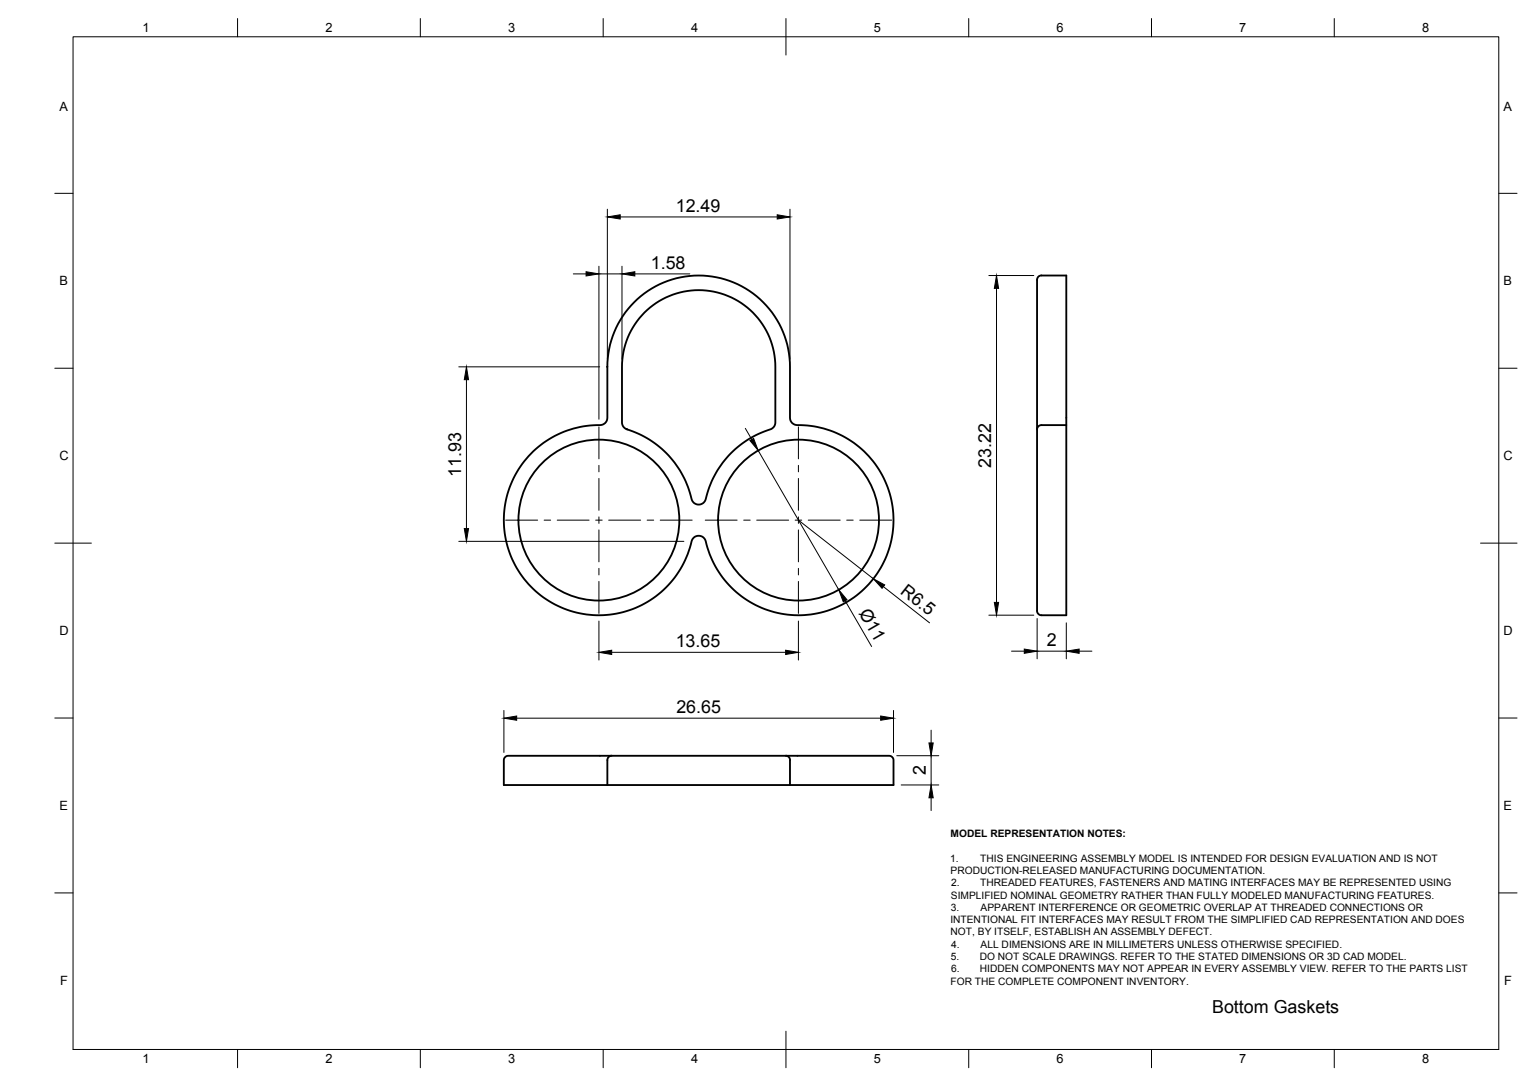
ISO-10303-21;
HEADER;
/* Generated by software containing ST-Developer
 * from STEP Tools, Inc. (www.steptools.com) 
 */

FILE_DESCRIPTION(
/* description */ ('STEP AP214'),
/* implementation_level */ '2;1');

FILE_NAME(
/* name */ 'Bottom Gaskets.step',
/* time_stamp */ '2026-10-06T00:19:40-07:00',
/* author */ (''),
/* organization */ (''),
/* preprocessor_version */ 'ST-DEVELOPER v20.2',
/* originating_system */ 'Autodesk Translation Framework v15.15.0.0',
/* authorisation */ '');

FILE_SCHEMA (('AUTOMOTIVE_DESIGN { 1 0 10303 214 3 1 1 }'));
ENDSEC;

DATA;
#10=MECHANICAL_DESIGN_GEOMETRIC_PRESENTATION_REPRESENTATION('',(#2066),#98302);
#118=TOROIDAL_SURFACE('',#34927,5.8,0.3);
#119=TOROIDAL_SURFACE('',#34931,5.8,0.3);
#569=ELLIPSE('',#34935,0.298848919318477,0.296905424707719);
#570=ELLIPSE('',#34936,0.298848892580485,0.296905360939291);
#571=ELLIPSE('',#34940,0.298848920090728,0.296905426638253);
#572=ELLIPSE('',#34941,0.29884889341624,0.296905361759044);
#573=ELLIPSE('',#34943,0.298848922260772,0.296905431625149);
#574=ELLIPSE('',#34945,0.298848920759339,0.296905428089205);
#575=ELLIPSE('',#34946,0.29884891933117,0.296905424743563);
#576=ELLIPSE('',#34947,0.298848915871755,0.296905416638318);
#577=ELLIPSE('',#34948,0.298848919843559,0.296905425953451);
#578=ELLIPSE('',#34949,0.298848891288725,0.296905359078035);
#579=ELLIPSE('',#34950,0.298848918410882,0.296905426718576);
#580=ELLIPSE('',#34951,0.298848922900226,0.296905433124464);
#581=ELLIPSE('',#34952,0.298848913927389,0.296905412076352);
#582=ELLIPSE('',#34953,0.298848922234263,0.296905431565699);
#583=ELLIPSE('',#34954,0.298848922236084,0.296905431557407);
#584=ELLIPSE('',#34956,0.298848891608559,0.296905359578392);
#585=ELLIPSE('',#34958,0.298848942238611,0.296905478386828);
#586=ELLIPSE('',#34959,0.298848922236084,0.296905431557407);
#1076=B_SPLINE_SURFACE_WITH_KNOTS('',5,5,((#72928,#72929,#72930,#72931,
#72932,#72933),(#72934,#72935,#72936,#72937,#72938,#72939),(#72940,#72941,
#72942,#72943,#72944,#72945),(#72946,#72947,#72948,#72949,#72950,#72951),
(#72952,#72953,#72954,#72955,#72956,#72957),(#72958,#72959,#72960,#72961,
#72962,#72963),(#72964,#72965,#72966,#72967,#72968,#72969),(#72970,#72971,
#72972,#72973,#72974,#72975),(#72976,#72977,#72978,#72979,#72980,#72981)),
 .UNSPECIFIED.,.F.,.F.,.F.,(6,3,6),(6,6),(0.546404786097,1.22269549144,
1.74380556781),(0.,0.3),.UNSPECIFIED.);
#1077=B_SPLINE_SURFACE_WITH_KNOTS('',5,1,((#72992,#72993),(#72994,#72995),
(#72996,#72997),(#72998,#72999),(#73000,#73001),(#73002,#73003)),
 .UNSPECIFIED.,.F.,.F.,.F.,(6,6),(2,2),(0.454732309483,1.10434989446),(0.,
0.204),.UNSPECIFIED.);
#1078=B_SPLINE_SURFACE_WITH_KNOTS('',5,5,((#73012,#73013,#73014,#73015,
#73016,#73017),(#73018,#73019,#73020,#73021,#73022,#73023),(#73024,#73025,
#73026,#73027,#73028,#73029),(#73030,#73031,#73032,#73033,#73034,#73035),
(#73036,#73037,#73038,#73039,#73040,#73041),(#73042,#73043,#73044,#73045,
#73046,#73047),(#73048,#73049,#73050,#73051,#73052,#73053),(#73054,#73055,
#73056,#73057,#73058,#73059),(#73060,#73061,#73062,#73063,#73064,#73065)),
 .UNSPECIFIED.,.F.,.F.,.F.,(6,3,6),(6,6),(6.80309055586,12.796423133,18.7900427979),
(0.,0.3),.UNSPECIFIED.);
#1079=B_SPLINE_SURFACE_WITH_KNOTS('',5,1,((#73074,#73075),(#73076,#73077),
(#73078,#73079),(#73080,#73081),(#73082,#73083),(#73084,#73085)),
 .UNSPECIFIED.,.F.,.F.,.F.,(6,6),(2,2),(5.9795921157,14.5218665667),(0.,
0.203999999999999),.UNSPECIFIED.);
#1080=B_SPLINE_SURFACE_WITH_KNOTS('',5,5,((#73087,#73088,#73089,#73090,
#73091,#73092),(#73093,#73094,#73095,#73096,#73097,#73098),(#73099,#73100,
#73101,#73102,#73103,#73104),(#73105,#73106,#73107,#73108,#73109,#73110),
(#73111,#73112,#73113,#73114,#73115,#73116),(#73117,#73118,#73119,#73120,
#73121,#73122),(#73123,#73124,#73125,#73126,#73127,#73128),(#73129,#73130,
#73131,#73132,#73133,#73134),(#73135,#73136,#73137,#73138,#73139,#73140)),
 .UNSPECIFIED.,.F.,.F.,.F.,(6,3,6),(6,6),(6.80400424079,13.5782854139,18.7904488943),
(0.,0.3),.UNSPECIFIED.);
#1081=B_SPLINE_SURFACE_WITH_KNOTS('',5,1,((#73201,#73202),(#73203,#73204),
(#73205,#73206),(#73207,#73208),(#73209,#73210),(#73211,#73212)),
 .UNSPECIFIED.,.F.,.F.,.F.,(6,6),(2,2),(5.9795921157,14.5218665667),(0.,
0.204),.UNSPECIFIED.);
#1082=B_SPLINE_SURFACE_WITH_KNOTS('',5,5,((#73220,#73221,#73222,#73223,
#73224,#73225),(#73226,#73227,#73228,#73229,#73230,#73231),(#73232,#73233,
#73234,#73235,#73236,#73237),(#73238,#73239,#73240,#73241,#73242,#73243),
(#73244,#73245,#73246,#73247,#73248,#73249),(#73250,#73251,#73252,#73253,
#73254,#73255),(#73256,#73257,#73258,#73259,#73260,#73261),(#73262,#73263,
#73264,#73265,#73266,#73267),(#73268,#73269,#73270,#73271,#73272,#73273)),
 .UNSPECIFIED.,.F.,.F.,.F.,(6,3,6),(6,6),(0.54640511867,1.22269582402,1.74380590038),
(0.,0.3),.UNSPECIFIED.);
#1083=B_SPLINE_SURFACE_WITH_KNOTS('',5,1,((#73282,#73283),(#73284,#73285),
(#73286,#73287),(#73288,#73289),(#73290,#73291),(#73292,#73293)),
 .UNSPECIFIED.,.F.,.F.,.F.,(6,6),(2,2),(0.454732309483,1.10434989446),(0.,
0.203999999999999),.UNSPECIFIED.);
#1084=B_SPLINE_SURFACE_WITH_KNOTS('',5,5,((#73295,#73296,#73297,#73298,
#73299,#73300),(#73301,#73302,#73303,#73304,#73305,#73306),(#73307,#73308,
#73309,#73310,#73311,#73312),(#73313,#73314,#73315,#73316,#73317,#73318),
(#73319,#73320,#73321,#73322,#73323,#73324),(#73325,#73326,#73327,#73328,
#73329,#73330),(#73331,#73332,#73333,#73334,#73335,#73336),(#73337,#73338,
#73339,#73340,#73341,#73342),(#73343,#73344,#73345,#73346,#73347,#73348)),
 .UNSPECIFIED.,.F.,.F.,.F.,(6,3,6),(6,6),(5.54615686267,10.8163068596,14.9229845471),
(0.,0.3),.UNSPECIFIED.);
#1085=B_SPLINE_SURFACE_WITH_KNOTS('',5,1,((#73357,#73358),(#73359,#73360),
(#73361,#73362),(#73363,#73364),(#73365,#73366),(#73367,#73368)),
 .UNSPECIFIED.,.F.,.F.,.F.,(6,6),(2,2),(4.82544286935,11.7189326827),(0.,
0.203999999999999),.UNSPECIFIED.);
#1086=B_SPLINE_SURFACE_WITH_KNOTS('',5,5,((#73370,#73371,#73372,#73373,
#73374,#73375),(#73376,#73377,#73378,#73379,#73380,#73381),(#73382,#73383,
#73384,#73385,#73386,#73387),(#73388,#73389,#73390,#73391,#73392,#73393),
(#73394,#73395,#73396,#73397,#73398,#73399),(#73400,#73401,#73402,#73403,
#73404,#73405),(#73406,#73407,#73408,#73409,#73410,#73411),(#73412,#73413,
#73414,#73415,#73416,#73417),(#73418,#73419,#73420,#73421,#73422,#73423)),
 .UNSPECIFIED.,.F.,.F.,.F.,(6,3,6),(6,6),(1.16471317114,2.5069575699,3.70327394785),
(0.,0.3),.UNSPECIFIED.);
#1087=B_SPLINE_SURFACE_WITH_KNOTS('',5,1,((#73478,#73479),(#73480,#73481),
(#73482,#73483),(#73484,#73485),(#73486,#73487),(#73488,#73489)),
 .UNSPECIFIED.,.F.,.F.,.F.,(6,6),(2,2),(1.04539060089,2.53880574503),(0.,
0.204),.UNSPECIFIED.);
#1088=B_SPLINE_SURFACE_WITH_KNOTS('',5,5,((#73491,#73492,#73493,#73494,
#73495,#73496),(#73497,#73498,#73499,#73500,#73501,#73502),(#73503,#73504,
#73505,#73506,#73507,#73508),(#73509,#73510,#73511,#73512,#73513,#73514),
(#73515,#73516,#73517,#73518,#73519,#73520),(#73521,#73522,#73523,#73524,
#73525,#73526),(#73527,#73528,#73529,#73530,#73531,#73532),(#73533,#73534,
#73535,#73536,#73537,#73538),(#73539,#73540,#73541,#73542,#73543,#73544)),
 .UNSPECIFIED.,.F.,.F.,.F.,(6,3,6),(6,6),(5.54628902772,10.8164390246,14.9231167121),
(0.,0.3),.UNSPECIFIED.);
#1089=B_SPLINE_SURFACE_WITH_KNOTS('',5,1,((#73551,#73552),(#73553,#73554),
(#73555,#73556),(#73557,#73558),(#73559,#73560),(#73561,#73562)),
 .UNSPECIFIED.,.F.,.F.,.F.,(6,6),(2,2),(4.82544286935,11.7189326827),(0.,
0.204),.UNSPECIFIED.);
#1090=B_SPLINE_SURFACE_WITH_KNOTS('',5,5,((#73563,#73564,#73565,#73566,
#73567,#73568),(#73569,#73570,#73571,#73572,#73573,#73574),(#73575,#73576,
#73577,#73578,#73579,#73580),(#73581,#73582,#73583,#73584,#73585,#73586),
(#73587,#73588,#73589,#73590,#73591,#73592),(#73593,#73594,#73595,#73596,
#73597,#73598),(#73599,#73600,#73601,#73602,#73603,#73604),(#73605,#73606,
#73607,#73608,#73609,#73610),(#73611,#73612,#73613,#73614,#73615,#73616)),
 .UNSPECIFIED.,.F.,.F.,.F.,(6,3,6),(6,6),(0.68208121853,1.52935115459,2.17454139046),
(0.,0.3),.UNSPECIFIED.);
#1091=B_SPLINE_SURFACE_WITH_KNOTS('',5,1,((#73627,#73628),(#73629,#73630),
(#73631,#73632),(#73633,#73634),(#73635,#73636),(#73637,#73638)),
 .UNSPECIFIED.,.F.,.F.,.F.,(6,6),(2,2),(0.574089330078,1.39421694447),(0.,
0.203999999999999),.UNSPECIFIED.);
#1092=B_SPLINE_SURFACE_WITH_KNOTS('',5,5,((#73641,#73642,#73643,#73644,
#73645,#73646),(#73647,#73648,#73649,#73650,#73651,#73652),(#73653,#73654,
#73655,#73656,#73657,#73658),(#73659,#73660,#73661,#73662,#73663,#73664),
(#73665,#73666,#73667,#73668,#73669,#73670),(#73671,#73672,#73673,#73674,
#73675,#73676),(#73677,#73678,#73679,#73680,#73681,#73682),(#73683,#73684,
#73685,#73686,#73687,#73688),(#73689,#73690,#73691,#73692,#73693,#73694),
(#73695,#73696,#73697,#73698,#73699,#73700),(#73701,#73702,#73703,#73704,
#73705,#73706),(#73707,#73708,#73709,#73710,#73711,#73712),(#73713,#73714,
#73715,#73716,#73717,#73718),(#73719,#73720,#73721,#73722,#73723,#73724),
(#73725,#73726,#73727,#73728,#73729,#73730)),.UNSPECIFIED.,.F.,.F.,.F.,
(6,3,3,3,6),(6,6),(13.4402611449,23.5689081291,33.6443676545,43.7196576595,
53.84849829),(0.,0.3),.UNSPECIFIED.);
#1093=B_SPLINE_SURFACE_WITH_KNOTS('',5,1,((#73748,#73749),(#73750,#73751),
(#73752,#73753),(#73754,#73755),(#73756,#73757),(#73758,#73759),(#73760,
#73761),(#73762,#73763),(#73764,#73765),(#73766,#73767),(#73768,#73769),
(#73770,#73771),(#73772,#73773),(#73774,#73775),(#73776,#73777)),
 .UNSPECIFIED.,.F.,.F.,.F.,(6,3,3,3,6),(2,2),(9.75975111992,17.2672519814,
24.7747528429,32.2822537043,39.7897545658),(0.,0.203999999999999),
 .UNSPECIFIED.);
#1094=B_SPLINE_SURFACE_WITH_KNOTS('',5,5,((#73779,#73780,#73781,#73782,
#73783,#73784),(#73785,#73786,#73787,#73788,#73789,#73790),(#73791,#73792,
#73793,#73794,#73795,#73796),(#73797,#73798,#73799,#73800,#73801,#73802),
(#73803,#73804,#73805,#73806,#73807,#73808),(#73809,#73810,#73811,#73812,
#73813,#73814),(#73815,#73816,#73817,#73818,#73819,#73820),(#73821,#73822,
#73823,#73824,#73825,#73826),(#73827,#73828,#73829,#73830,#73831,#73832)),
 .UNSPECIFIED.,.F.,.F.,.F.,(6,3,6),(6,6),(0.578957415869,1.29652194364,
1.84813902128),(0.,0.3),.UNSPECIFIED.);
#1095=B_SPLINE_SURFACE_WITH_KNOTS('',5,1,((#73841,#73842),(#73843,#73844),
(#73845,#73846),(#73847,#73848),(#73849,#73850),(#73851,#73852)),
 .UNSPECIFIED.,.F.,.F.,.F.,(6,6),(2,2),(0.48312294093,1.17329857083),(0.,
0.203999999999999),.UNSPECIFIED.);
#1096=B_SPLINE_SURFACE_WITH_KNOTS('',5,5,((#73854,#73855,#73856,#73857,
#73858,#73859),(#73860,#73861,#73862,#73863,#73864,#73865),(#73866,#73867,
#73868,#73869,#73870,#73871),(#73872,#73873,#73874,#73875,#73876,#73877),
(#73878,#73879,#73880,#73881,#73882,#73883),(#73884,#73885,#73886,#73887,
#73888,#73889),(#73890,#73891,#73892,#73893,#73894,#73895),(#73896,#73897,
#73898,#73899,#73900,#73901),(#73902,#73903,#73904,#73905,#73906,#73907)),
 .UNSPECIFIED.,.F.,.F.,.F.,(6,3,6),(6,6),(0.579418789984,1.29713059772,
1.84860050261),(0.,0.3),.UNSPECIFIED.);
#1097=B_SPLINE_SURFACE_WITH_KNOTS('',5,1,((#73916,#73917),(#73918,#73919),
(#73920,#73921),(#73922,#73923),(#73924,#73925),(#73926,#73927)),
 .UNSPECIFIED.,.F.,.F.,.F.,(6,6),(2,2),(0.48312294093,1.17329857083),(0.,
0.204),.UNSPECIFIED.);
#1098=B_SPLINE_SURFACE_WITH_KNOTS('',5,5,((#73929,#73930,#73931,#73932,
#73933,#73934),(#73935,#73936,#73937,#73938,#73939,#73940),(#73941,#73942,
#73943,#73944,#73945,#73946),(#73947,#73948,#73949,#73950,#73951,#73952),
(#73953,#73954,#73955,#73956,#73957,#73958),(#73959,#73960,#73961,#73962,
#73963,#73964),(#73965,#73966,#73967,#73968,#73969,#73970),(#73971,#73972,
#73973,#73974,#73975,#73976),(#73977,#73978,#73979,#73980,#73981,#73982),
(#73983,#73984,#73985,#73986,#73987,#73988),(#73989,#73990,#73991,#73992,
#73993,#73994),(#73995,#73996,#73997,#73998,#73999,#74000),(#74001,#74002,
#74003,#74004,#74005,#74006),(#74007,#74008,#74009,#74010,#74011,#74012),
(#74013,#74014,#74015,#74016,#74017,#74018)),.UNSPECIFIED.,.F.,.F.,.F.,
(6,3,3,3,6),(6,6),(13.4404181035,23.5157081046,33.5961540362,43.6766373031,
53.8487877185),(0.,0.3),.UNSPECIFIED.);
#1099=B_SPLINE_SURFACE_WITH_KNOTS('',5,1,((#74036,#74037),(#74038,#74039),
(#74040,#74041),(#74042,#74043),(#74044,#74045),(#74046,#74047),(#74048,
#74049),(#74050,#74051),(#74052,#74053),(#74054,#74055),(#74056,#74057),
(#74058,#74059),(#74060,#74061),(#74062,#74063),(#74064,#74065)),
 .UNSPECIFIED.,.F.,.F.,.F.,(6,3,3,3,6),(2,2),(9.75975111992,17.2672519814,
24.7747528429,32.2822537043,39.7897545658),(0.,0.203999999999999),
 .UNSPECIFIED.);
#1100=B_SPLINE_SURFACE_WITH_KNOTS('',5,5,((#74067,#74068,#74069,#74070,
#74071,#74072),(#74073,#74074,#74075,#74076,#74077,#74078),(#74079,#74080,
#74081,#74082,#74083,#74084),(#74085,#74086,#74087,#74088,#74089,#74090),
(#74091,#74092,#74093,#74094,#74095,#74096),(#74097,#74098,#74099,#74100,
#74101,#74102),(#74103,#74104,#74105,#74106,#74107,#74108),(#74109,#74110,
#74111,#74112,#74113,#74114),(#74115,#74116,#74117,#74118,#74119,#74120)),
 .UNSPECIFIED.,.F.,.F.,.F.,(6,3,6),(6,6),(0.682080632107,1.52935056816,
2.17454080403),(0.,0.3),.UNSPECIFIED.);
#1101=B_SPLINE_SURFACE_WITH_KNOTS('',5,1,((#74129,#74130),(#74131,#74132),
(#74133,#74134),(#74135,#74136),(#74137,#74138),(#74139,#74140)),
 .UNSPECIFIED.,.F.,.F.,.F.,(6,6),(2,2),(0.574089330078,1.39421694447),(0.,
0.203999999999999),.UNSPECIFIED.);
#1102=B_SPLINE_SURFACE_WITH_KNOTS('',5,5,((#74148,#74149,#74150,#74151,
#74152,#74153),(#74154,#74155,#74156,#74157,#74158,#74159),(#74160,#74161,
#74162,#74163,#74164,#74165),(#74166,#74167,#74168,#74169,#74170,#74171),
(#74172,#74173,#74174,#74175,#74176,#74177),(#74178,#74179,#74180,#74181,
#74182,#74183),(#74184,#74185,#74186,#74187,#74188,#74189),(#74190,#74191,
#74192,#74193,#74194,#74195),(#74196,#74197,#74198,#74199,#74200,#74201)),
 .UNSPECIFIED.,.F.,.F.,.F.,(6,3,6),(6,6),(8.03777014773,13.7697600959,21.5792812917),
(0.,0.3),.UNSPECIFIED.);
#1103=B_SPLINE_SURFACE_WITH_KNOTS('',5,1,((#74210,#74211),(#74212,#74213),
(#74214,#74215),(#74216,#74217),(#74218,#74219),(#74220,#74221)),
 .UNSPECIFIED.,.F.,.F.,.F.,(6,6),(2,2),(7.11986732816,17.2911063684),(0.,
0.204),.UNSPECIFIED.);
#1104=B_SPLINE_SURFACE_WITH_KNOTS('',5,5,((#74223,#74224,#74225,#74226,
#74227,#74228),(#74229,#74230,#74231,#74232,#74233,#74234),(#74235,#74236,
#74237,#74238,#74239,#74240),(#74241,#74242,#74243,#74244,#74245,#74246),
(#74247,#74248,#74249,#74250,#74251,#74252),(#74253,#74254,#74255,#74256,
#74257,#74258),(#74259,#74260,#74261,#74262,#74263,#74264),(#74265,#74266,
#74267,#74268,#74269,#74270),(#74271,#74272,#74273,#74274,#74275,#74276)),
 .UNSPECIFIED.,.F.,.F.,.F.,(6,3,6),(6,6),(8.03689290773,13.768506892,21.5784150656),
(0.,0.3),.UNSPECIFIED.);
#1105=B_SPLINE_SURFACE_WITH_KNOTS('',5,1,((#74285,#74286),(#74287,#74288),
(#74289,#74290),(#74291,#74292),(#74293,#74294),(#74295,#74296)),
 .UNSPECIFIED.,.F.,.F.,.F.,(6,6),(2,2),(7.11986732816,17.2911063684),(0.,
0.204000000000001),.UNSPECIFIED.);
#1268=FACE_BOUND('',#5840,.T.);
#1269=FACE_BOUND('',#5841,.T.);
#1270=FACE_BOUND('',#5842,.T.);
#1271=FACE_BOUND('',#5844,.T.);
#1272=FACE_BOUND('',#5845,.T.);
#1273=FACE_BOUND('',#5846,.T.);
#1591=B_SPLINE_CURVE_WITH_KNOTS('',3,(#71744,#71745,#71746,#71747,#71748,
#71749,#71750,#71751,#71752,#71753,#71754,#71755,#71756,#71757,#71758,#71759,
#71760,#71761,#71762,#71763,#71764,#71765,#71766,#71767,#71768,#71769,#71770,
#71771,#71772,#71773,#71774,#71775,#71776,#71777,#71778,#71779,#71780,#71781,
#71782,#71783,#71784,#71785,#71786,#71787,#71788,#71789,#71790,#71791,#71792,
#71793,#71794,#71795,#71796,#71797,#71798,#71799,#71800,#71801,#71802,#71803,
#71804,#71805,#71806,#71807,#71808,#71809,#71810,#71811,#71812,#71813,#71814,
#71815,#71816,#71817,#71818,#71819,#71820,#71821,#71822,#71823,#71824,#71825,
#71826,#71827,#71828,#71829,#71830,#71831,#71832,#71833,#71834,#71835,#71836,
#71837,#71838,#71839,#71840,#71841,#71842,#71843,#71844,#71845,#71846,#71847,
#71848,#71849,#71850,#71851,#71852,#71853,#71854,#71855,#71856,#71857,#71858,
#71859,#71860,#71861,#71862,#71863,#71864,#71865,#71866,#71867,#71868,#71869,
#71870,#71871,#71872,#71873,#71874,#71875,#71876,#71877,#71878,#71879,#71880,
#71881,#71882,#71883,#71884,#71885,#71886,#71887,#71888,#71889,#71890,#71891,
#71892,#71893,#71894,#71895,#71896,#71897,#71898,#71899,#71900,#71901,#71902,
#71903,#71904,#71905,#71906,#71907,#71908,#71909,#71910,#71911,#71912,#71913,
#71914,#71915,#71916,#71917,#71918),.UNSPECIFIED.,.F.,.F.,(4,3,3,3,3,3,
3,3,3,3,3,3,3,3,3,3,3,3,3,3,3,3,3,3,3,3,3,3,3,3,3,3,3,3,3,3,3,3,3,3,3,3,
3,3,3,3,3,3,3,3,3,3,3,3,3,3,3,3,4),(13.4402611449,13.5070964098,14.2468335688477,
14.9953689393349,15.7485030377147,16.5054819020246,17.2654067660921,18.0278474779116,
18.7905126436479,19.5517539434494,20.2095273779,20.9687643902614,21.7217135386243,
22.4703077255754,23.2116440479358,23.5689081291,24.3109067601058,25.0584792099068,
25.8110233837674,26.567773191108,27.3278022892921,28.1173729599431,28.8763863467288,
29.6393660388709,30.4006119455066,31.159144897169,31.9121345408492,32.6611814951464,
33.4038368880882,33.6443676545,34.3873867942773,35.135806909375,35.888999131998,
36.6461739203357,37.4063879012094,38.1955466209957,38.955487589057,39.7175566740638,
40.477710487504,41.2350068233562,41.9866165086,42.7342388949353,43.4754422745138,
43.7196576595,44.4613265079885,45.2089180014669,45.9618189072157,46.719235518721,
47.4801950110937,48.2678785133445,49.0291748631258,49.7910234685431,50.5510731777613,
51.3083055012999,52.0598033404119,52.8072294015329,53.5481010611059,53.7816630291,
53.84849829),.UNSPECIFIED.);
#1592=B_SPLINE_CURVE_WITH_KNOTS('',3,(#71920,#71921,#71922,#71923,#71924,
#71925,#71926,#71927,#71928,#71929,#71930,#71931,#71932,#71933,#71934,#71935,
#71936,#71937,#71938,#71939,#71940,#71941,#71942,#71943,#71944,#71945,#71946,
#71947,#71948,#71949,#71950,#71951,#71952,#71953,#71954,#71955,#71956,#71957,
#71958,#71959,#71960,#71961,#71962,#71963,#71964,#71965),.UNSPECIFIED.,
 .F.,.F.,(4,3,3,3,3,3,3,3,3,3,3,3,3,3,3,4),(0.68208121853,0.833285110291927,
0.893438704333,1.03975468193142,1.10556304245,1.23772138518436,1.36639838409707,
1.49153340548065,1.52935115459,1.66108737747387,1.74128259681,1.88383305622587,
1.95314956045,2.12228973264587,2.16523839884,2.17454139046),
 .UNSPECIFIED.);
#1593=B_SPLINE_CURVE_WITH_KNOTS('',3,(#71969,#71970,#71971,#71972,#71973,
#71974,#71975,#71976,#71977,#71978,#71979,#71980,#71981,#71982,#71983,#71984,
#71985,#71986,#71987,#71988,#71989,#71990,#71991,#71992,#71993,#71994,#71995,
#71996,#71997,#71998,#71999,#72000,#72001,#72002,#72003,#72004,#72005,#72006,
#72007,#72008,#72009,#72010,#72011,#72012,#72013,#72014,#72015,#72016,#72017,
#72018,#72019,#72020,#72021,#72022,#72023,#72024,#72025,#72026,#72027,#72028,
#72029),.UNSPECIFIED.,.F.,.F.,(4,3,3,3,3,3,3,3,3,3,3,3,3,3,3,3,3,3,3,3,
4),(8.03689290773,8.75334465576375,9.46923125712186,10.1895756567313,10.9140328563649,
11.6440191235026,12.3764813091007,13.1119708062231,13.768506892,14.5052662832091,
15.243807631294,15.9828982697244,16.7204464834581,17.4556667504414,18.1876202191916,
18.9154953869,19.6359475654664,20.3517214078531,21.0597384561033,21.5454531764,
21.5784150656),.UNSPECIFIED.);
#1594=B_SPLINE_CURVE_WITH_KNOTS('',3,(#72031,#72032,#72033,#72034,#72035,
#72036,#72037,#72038,#72039,#72040,#72041,#72042,#72043,#72044,#72045,#72046,
#72047,#72048,#72049,#72050,#72051,#72052,#72053,#72054,#72055,#72056,#72057,
#72058,#72059,#72060,#72061,#72062,#72063,#72064,#72065,#72066,#72067,#72068,
#72069,#72070,#72071,#72072,#72073,#72074,#72075,#72076,#72077,#72078,#72079,
#72080,#72081,#72082,#72083,#72084,#72085,#72086,#72087,#72088,#72089,#72090,
#72091),.UNSPECIFIED.,.F.,.F.,(4,3,3,3,3,3,3,3,3,3,3,3,3,3,3,3,3,3,3,3,
4),(8.03777014773,8.75426889125125,9.47001359609466,10.1902177205057,10.9145366724205,
11.6443893801527,12.3767202822979,13.1120832966385,13.7697600959,14.5065337688577,
15.2451024323911,15.9842354518727,16.7218509387113,17.4571540774596,18.1892052935327,
18.9171918235122,19.6377739811748,20.3536859093427,21.0618537376259,21.5465332101,
21.5792812917),.UNSPECIFIED.);
#1595=B_SPLINE_CURVE_WITH_KNOTS('',3,(#72095,#72096,#72097,#72098,#72099,
#72100,#72101,#72102,#72103,#72104,#72105,#72106,#72107,#72108,#72109,#72110,
#72111,#72112,#72113,#72114,#72115,#72116,#72117,#72118,#72119,#72120,#72121,
#72122,#72123,#72124,#72125,#72126,#72127,#72128,#72129,#72130,#72131,#72132,
#72133,#72134,#72135,#72136,#72137,#72138,#72139,#72140),.UNSPECIFIED.,
 .F.,.F.,(4,3,3,3,3,3,3,3,3,3,3,3,3,3,3,4),(0.682080632107,0.833188271917978,
0.893438117902,1.03975409805662,1.10556245601,1.23772079875137,1.36639779750311,
1.49153281928841,1.52935056816,1.66108679248608,1.74128201038,1.88383247191979,
1.95314897402,2.12228914750544,2.16523781241,2.17454080403),
 .UNSPECIFIED.);
#1596=B_SPLINE_CURVE_WITH_KNOTS('',3,(#72142,#72143,#72144,#72145,#72146,
#72147,#72148,#72149,#72150,#72151,#72152,#72153,#72154,#72155,#72156,#72157,
#72158,#72159,#72160,#72161,#72162,#72163,#72164,#72165,#72166,#72167,#72168,
#72169,#72170,#72171,#72172,#72173,#72174,#72175,#72176,#72177,#72178,#72179,
#72180,#72181,#72182,#72183,#72184,#72185,#72186,#72187,#72188,#72189,#72190,
#72191,#72192,#72193,#72194,#72195,#72196,#72197,#72198,#72199,#72200,#72201,
#72202,#72203,#72204,#72205,#72206,#72207,#72208,#72209,#72210,#72211,#72212,
#72213,#72214,#72215,#72216,#72217,#72218,#72219,#72220,#72221,#72222,#72223,
#72224,#72225,#72226,#72227,#72228,#72229,#72230,#72231,#72232,#72233,#72234,
#72235,#72236,#72237,#72238,#72239,#72240,#72241,#72242,#72243,#72244,#72245,
#72246,#72247,#72248,#72249,#72250,#72251,#72252,#72253,#72254,#72255,#72256,
#72257,#72258,#72259,#72260,#72261,#72262,#72263,#72264,#72265,#72266,#72267,
#72268,#72269,#72270,#72271,#72272,#72273,#72274,#72275,#72276,#72277,#72278,
#72279,#72280,#72281,#72282,#72283,#72284,#72285,#72286,#72287,#72288,#72289,
#72290,#72291,#72292,#72293,#72294,#72295,#72296,#72297,#72298,#72299,#72300,
#72301,#72302,#72303,#72304,#72305,#72306,#72307,#72308,#72309,#72310,#72311,
#72312,#72313),.UNSPECIFIED.,.F.,.F.,(4,3,3,3,3,3,3,3,3,3,3,3,3,3,3,3,3,
3,3,3,3,3,3,3,3,3,3,3,3,3,3,3,3,3,3,3,3,3,3,3,3,3,3,3,3,3,3,3,3,3,3,3,3,
3,3,3,3,4),(13.4404181035,14.1832469713423,14.9311788451456,15.6836632577811,
16.4417307823792,17.202055740606,17.9644513437534,18.4746549323,19.2374710902407,
19.9985815368466,20.7569924140862,21.509630605407,22.2582851244697,22.9999062408337,
23.5157081046,24.2597621045338,25.0092545320489,25.7635337985687,26.521784600003,
27.2830357102544,28.0721755009976,28.8305221896519,29.5929229482329,30.3533096498532,
31.1107361457363,31.8623257075202,32.6098454986528,33.3508338437457,33.5961540362,
34.3408789768401,35.0909966454356,35.8458336275569,36.6045522537918,37.3661601097332,
38.154969758904,38.8368239887457,39.599089755228,40.3593159984205,41.116556848427,
41.8678616724636,42.6150717427155,43.3555578410029,43.6766373031,44.4154372840554,
45.1632743442511,45.9157419950385,46.6741354613049,47.0360646138,47.7955806316773,
48.5576994151819,49.3198406379445,50.0808007763051,50.839431318698,51.5923911750364,
52.3413609598882,53.0826832013661,53.8176639786,53.8487877185),
 .UNSPECIFIED.);
#1597=B_SPLINE_CURVE_WITH_KNOTS('',3,(#72315,#72316,#72317,#72318,#72319,
#72320,#72321,#72322,#72323,#72324,#72325,#72326,#72327,#72328,#72329,#72330,
#72331,#72332,#72333,#72334,#72335,#72336,#72337,#72338,#72339,#72340,#72341,
#72342,#72343,#72344,#72345,#72346,#72347,#72348,#72349,#72350,#72351,#72352,
#72353,#72354),.UNSPECIFIED.,.F.,.F.,(4,3,3,3,3,3,3,3,3,3,3,3,3,4),(0.579418789984,
0.725653581578792,0.867122312367032,0.938068556291,1.07176782281773,1.11759224819,
1.24463101759673,1.29713059772,1.42927287787526,1.47665930895,1.61898723804258,
1.77132177608973,1.83573111331,1.84860050261),.UNSPECIFIED.);
#1598=B_SPLINE_CURVE_WITH_KNOTS('',3,(#72355,#72356,#72357,#72358,#72359,
#72360,#72361,#72362,#72363,#72364,#72365,#72366,#72367,#72368,#72369,#72370,
#72371,#72372,#72373,#72374,#72375,#72376,#72377,#72378,#72379,#72380,#72381,
#72382,#72383,#72384,#72385,#72386,#72387,#72388,#72389,#72390,#72391,#72392,
#72393,#72394),.UNSPECIFIED.,.F.,.F.,(4,3,3,3,3,3,3,3,3,3,3,3,3,4),(0.578957415869,
0.726935642898053,0.869358464457875,0.937512229109,1.07080769681197,1.19853817927595,
1.29652194364,1.42846234265899,1.4760627343,1.61769834304174,1.76863899687797,
1.83522042146,1.84649047214,1.84813902128),.UNSPECIFIED.);
#1599=B_SPLINE_CURVE_WITH_KNOTS('',3,(#72399,#72400,#72401,#72402,#72403,
#72404,#72405,#72406,#72407,#72408,#72409,#72410,#72411,#72412,#72413,#72414,
#72415,#72416,#72417,#72418,#72419,#72420,#72421,#72422,#72423,#72424,#72425,
#72426,#72427,#72428,#72429,#72430,#72431,#72432,#72433,#72434,#72435,#72436,
#72437,#72438),.UNSPECIFIED.,.F.,.F.,(4,3,3,3,3,3,3,3,3,3,3,3,3,4),(0.546404786097,
0.691378490918164,0.831851442486203,0.884338413692,1.0179759898933,1.05350843186,
1.1812184524978,1.22269549144,1.35451436280229,1.49122152065914,1.56106898317,
1.71044921676803,1.74092276094,1.74380556781),.UNSPECIFIED.);
#1600=B_SPLINE_CURVE_WITH_KNOTS('',3,(#72440,#72441,#72442,#72443,#72444,
#72445,#72446,#72447,#72448,#72449,#72450,#72451,#72452,#72453,#72454,#72455,
#72456,#72457,#72458,#72459,#72460,#72461,#72462,#72463,#72464,#72465,#72466,
#72467,#72468,#72469,#72470,#72471,#72472,#72473,#72474,#72475,#72476,#72477,
#72478,#72479,#72480,#72481,#72482),.UNSPECIFIED.,.F.,.F.,(4,3,3,3,3,3,
3,3,3,3,3,3,3,3,4),(5.54628902772,6.33044435630308,7.10830578793151,7.87994882881436,
8.64217889818713,9.39932532520428,10.1484181785832,10.8164390246,11.563804771993,
12.3219342993112,13.0975455758633,13.8843705850609,14.6884227142447,14.8537077686,
14.9231167121),.UNSPECIFIED.);
#1601=B_SPLINE_CURVE_WITH_KNOTS('',3,(#72484,#72485,#72486,#72487,#72488,
#72489,#72490,#72491,#72492,#72493,#72494,#72495,#72496,#72497,#72498,#72499,
#72500,#72501,#72502,#72503,#72504,#72505,#72506,#72507,#72508,#72509,#72510,
#72511,#72512,#72513,#72514,#72515,#72516,#72517,#72518,#72519,#72520,#72521,
#72522,#72523,#72524,#72525,#72526,#72527,#72528,#72529,#72530,#72531,#72532,
#72533,#72534,#72535,#72536,#72537,#72538,#72539,#72540,#72541,#72542,#72543,
#72544,#72545,#72546,#72547,#72548,#72549,#72550,#72551,#72552,#72553,#72554,
#72555,#72556,#72557,#72558,#72559),.UNSPECIFIED.,.F.,.F.,(4,3,3,3,3,3,
3,3,3,3,3,3,3,3,3,3,3,3,3,3,3,3,3,3,3,4),(1.16471317114,1.28955678457906,
1.34495894511,1.4697639644744,1.52520817925,1.65292971547884,1.76872520496,
1.90134001405299,2.0346343138382,2.13573896786,2.26681625793335,2.39531374620892,
2.5069575699,2.6339538548235,2.76351336933892,2.87774629091,3.00835142684093,
3.12090556789,3.24957903139955,3.30443948601,3.43081011387895,3.48797183209,
3.613503668297,3.67393178216,3.69717524887,3.70327394785),.UNSPECIFIED.);
#1602=B_SPLINE_CURVE_WITH_KNOTS('',3,(#72561,#72562,#72563,#72564,#72565,
#72566,#72567,#72568,#72569,#72570,#72571,#72572,#72573,#72574,#72575,#72576,
#72577,#72578,#72579,#72580,#72581,#72582,#72583,#72584,#72585,#72586,#72587,
#72588,#72589,#72590,#72591,#72592,#72593,#72594,#72595,#72596,#72597,#72598,
#72599,#72600,#72601,#72602,#72603,#72604,#72605,#72606),.UNSPECIFIED.,
 .F.,.F.,(4,3,3,3,3,3,3,3,3,3,3,3,3,3,3,4),(5.54615686267,6.33030620256032,
7.10816058979279,7.87979597471841,8.64201814773229,9.39915688584315,10.1482427247414,
10.8163068596,11.5638110745412,12.3220901845671,13.098030834098,13.8852098339371,
14.4040971905186,14.6843128354211,14.8776367646747,14.9229845471),
 .UNSPECIFIED.);
#1603=B_SPLINE_CURVE_WITH_KNOTS('',3,(#72608,#72609,#72610,#72611,#72612,
#72613,#72614,#72615,#72616,#72617,#72618,#72619,#72620,#72621,#72622,#72623,
#72624,#72625,#72626,#72627,#72628,#72629,#72630,#72631,#72632,#72633,#72634,
#72635,#72636,#72637,#72638,#72639,#72640,#72641,#72642,#72643,#72644),
 .UNSPECIFIED.,.F.,.F.,(4,3,3,3,3,3,3,3,3,3,3,3,4),(0.54640511867,0.69038189628902,
0.831066058366692,0.965751341507189,1.05350876443,1.1812187883191,1.22269582402,
1.35451469641816,1.49122185483681,1.56106931574,1.71044954193083,1.74092309351,
1.74380590038),.UNSPECIFIED.);
#1604=B_SPLINE_CURVE_WITH_KNOTS('',3,(#72648,#72649,#72650,#72651,#72652,
#72653,#72654,#72655,#72656,#72657,#72658,#72659,#72660,#72661,#72662,#72663,
#72664,#72665,#72666,#72667,#72668,#72669,#72670,#72671,#72672,#72673,#72674,
#72675,#72676,#72677,#72678,#72679,#72680,#72681,#72682,#72683,#72684,#72685,
#72686,#72687,#72688,#72689,#72690,#72691,#72692,#72693,#72694,#72695,#72696,
#72697,#72698,#72699,#72700,#72701,#72702,#72703,#72704,#72705,#72706,#72707,
#72708),.UNSPECIFIED.,.F.,.F.,(4,3,3,3,3,3,3,3,3,3,3,3,3,3,3,3,3,3,3,3,
4),(6.80400424079,7.43551608490868,8.07296241255818,8.71878211416777,9.36915323230095,
10.0253311081077,10.185707897,10.847851527524,11.530459999118,12.1974538393883,
12.8878696266442,13.5782854139,14.2435799397826,14.905962344532,15.5649203367182,
16.2200258486319,16.8684640346437,17.5129910403709,18.1507928771493,18.7732643273,
18.7904488943),.UNSPECIFIED.);
#1605=B_SPLINE_CURVE_WITH_KNOTS('',3,(#72709,#72710,#72711,#72712,#72713,
#72714,#72715,#72716,#72717,#72718,#72719,#72720,#72721,#72722,#72723,#72724,
#72725,#72726,#72727,#72728,#72729,#72730,#72731,#72732,#72733,#72734,#72735,
#72736,#72737,#72738,#72739,#72740,#72741,#72742,#72743,#72744,#72745,#72746,
#72747,#72748,#72749,#72750,#72751,#72752,#72753,#72754,#72755,#72756,#72757,
#72758,#72759,#72760,#72761,#72762,#72763,#72764,#72765,#72766,#72767,#72768,
#72769,#72770,#72771,#72772,#72773,#72774,#72775),.UNSPECIFIED.,.F.,.F.,
(4,3,3,3,3,3,3,3,3,3,3,3,3,3,3,3,3,3,3,3,3,3,4),(6.80309055586,6.83920298432,
7.47379817923227,8.13912629845323,8.78763073366937,9.44086248718233,10.0984392541387,
10.7729352238541,11.4388498023207,12.1176364676603,12.796423133,13.4656868144225,
14.132263549812,14.7961195641698,15.4565492516297,16.112959614828,16.782230410596,
17.4269097691535,18.0671355216093,18.4285891597547,18.6334246721777,18.7701216625788,
18.7900427979),.UNSPECIFIED.);
#1606=B_SPLINE_CURVE_WITH_KNOTS('',5,(#72783,#72784,#72785,#72786,#72787,
#72788),.UNSPECIFIED.,.F.,.F.,(6,6),(-0.791045523784,0.),.UNSPECIFIED.);
#1607=B_SPLINE_CURVE_WITH_KNOTS('',5,(#72790,#72791,#72792,#72793,#72794,
#72795,#72796,#72797,#72798,#72799,#72800,#72801,#72802,#72803,#72804),
 .UNSPECIFIED.,.F.,.F.,(6,3,3,3,6),(-30.0305934991,-22.7207065053,-15.4108195114,
-8.10093251761,-0.791045523784),.UNSPECIFIED.);
#1608=B_SPLINE_CURVE_WITH_KNOTS('',5,(#72806,#72807,#72808,#72809,#72810,
#72811),.UNSPECIFIED.,.F.,.F.,(6,6),(-30.70334581,-30.0305934991),
 .UNSPECIFIED.);
#1609=B_SPLINE_CURVE_WITH_KNOTS('',5,(#72813,#72814,#72815,#72816,#72817,
#72818),.UNSPECIFIED.,.F.,.F.,(6,6),(-31.3760981209,-30.70334581),
 .UNSPECIFIED.);
#1610=B_SPLINE_CURVE_WITH_KNOTS('',5,(#72820,#72821,#72822,#72823,#72824,
#72825,#72826,#72827,#72828,#72829,#72830,#72831,#72832,#72833,#72834),
 .UNSPECIFIED.,.F.,.F.,(6,3,3,3,6),(-60.6156460962,-53.3057591024,-45.9958721086,
-38.6859851147,-31.3760981209),.UNSPECIFIED.);
#1611=B_SPLINE_CURVE_WITH_KNOTS('',5,(#72836,#72837,#72838,#72839,#72840,
#72841),.UNSPECIFIED.,.F.,.F.,(6,6),(-61.40669162,-60.6156460962),
 .UNSPECIFIED.);
#1612=B_SPLINE_CURVE_WITH_KNOTS('',5,(#72845,#72846,#72847,#72848,#72849,
#72850),.UNSPECIFIED.,.F.,.F.,(6,6),(-74.6958207115,-64.888669513),
 .UNSPECIFIED.);
#1613=B_SPLINE_CURVE_WITH_KNOTS('',5,(#72852,#72853,#72854,#72855,#72856,
#72857),.UNSPECIFIED.,.F.,.F.,(6,6),(-84.5029719101,-74.6958207115),
 .UNSPECIFIED.);
#1614=B_SPLINE_CURVE_WITH_KNOTS('',5,(#72865,#72866,#72867,#72868,#72869,
#72870),.UNSPECIFIED.,.F.,.F.,(6,6),(0.,0.634618899121),.UNSPECIFIED.);
#1615=B_SPLINE_CURVE_WITH_KNOTS('',5,(#72874,#72875,#72876,#72877,#72878,
#72879),.UNSPECIFIED.,.F.,.F.,(6,6),(4.43202703274,12.6683819045),
 .UNSPECIFIED.);
#1616=B_SPLINE_CURVE_WITH_KNOTS('',5,(#72881,#72882,#72883,#72884,#72885,
#72886),.UNSPECIFIED.,.F.,.F.,(6,6),(12.6683819045,20.9047367763),
 .UNSPECIFIED.);
#1617=B_SPLINE_CURVE_WITH_KNOTS('',5,(#72890,#72891,#72892,#72893,#72894,
#72895),.UNSPECIFIED.,.F.,.F.,(6,6),(24.7021449099,25.336763809),
 .UNSPECIFIED.);
#1618=B_SPLINE_CURVE_WITH_KNOTS('',5,(#72897,#72898,#72899,#72900,#72901,
#72902),.UNSPECIFIED.,.F.,.F.,(6,6),(25.336763809,32.1215862286),
 .UNSPECIFIED.);
#1619=B_SPLINE_CURVE_WITH_KNOTS('',5,(#72904,#72905,#72906,#72907,#72908,
#72909),.UNSPECIFIED.,.F.,.F.,(6,6),(32.1215862286,33.4669635909),
 .UNSPECIFIED.);
#1620=B_SPLINE_CURVE_WITH_KNOTS('',5,(#72910,#72911,#72912,#72913,#72914,
#72915),.UNSPECIFIED.,.F.,.F.,(6,6),(33.4669635909,40.2517860105),
 .UNSPECIFIED.);
#1621=B_SPLINE_CURVE_WITH_KNOTS('',5,(#72986,#72987,#72988,#72989,#72990,
#72991),.UNSPECIFIED.,.F.,.F.,(6,6),(0.,1.),.UNSPECIFIED.);
#1622=B_SPLINE_CURVE_WITH_KNOTS('',5,(#73068,#73069,#73070,#73071,#73072,
#73073),.UNSPECIFIED.,.F.,.F.,(6,6),(4.43202703274,12.6683819045),
 .UNSPECIFIED.);
#1623=B_SPLINE_CURVE_WITH_KNOTS('',3,(#73143,#73144,#73145,#73146,#73147,
#73148,#73149,#73150,#73151,#73152,#73153,#73154,#73155,#73156,#73157,#73158,
#73159,#73160,#73161,#73162,#73163,#73164,#73165,#73166,#73167,#73168,#73169,
#73170,#73171,#73172,#73173,#73174,#73175,#73176,#73177,#73178,#73179,#73180,
#73181,#73182,#73183,#73184,#73185,#73186,#73187,#73188,#73189,#73190,#73191,
#73192,#73193,#73194,#73195,#73196,#73197,#73198,#73199,#73200),
 .UNSPECIFIED.,.F.,.F.,(4,3,3,3,3,3,3,3,3,3,3,3,3,3,3,3,3,3,3,4),(12.6683819045,
13.1106199615824,13.5570304890591,14.0277809275642,14.4835378398279,14.9420145479918,
15.4026526010081,15.882747950031,16.3457775995096,16.8085437495859,17.2700435239617,
17.3230339970997,17.7823518959161,18.2417043637307,18.7003769570558,19.1576865479113,
19.6116903525143,20.0633375875012,20.5105511785383,20.9047367763),
 .UNSPECIFIED.);
#1624=B_SPLINE_CURVE_WITH_KNOTS('',5,(#73276,#73277,#73278,#73279,#73280,
#73281),.UNSPECIFIED.,.F.,.F.,(6,6),(0.,1.),.UNSPECIFIED.);
#1625=B_SPLINE_CURVE_WITH_KNOTS('',5,(#73351,#73352,#73353,#73354,#73355,
#73356),.UNSPECIFIED.,.F.,.F.,(6,6),(25.336763809,32.1215862286),
 .UNSPECIFIED.);
#1626=B_SPLINE_CURVE_WITH_KNOTS('',3,(#73426,#73427,#73428,#73429,#73430,
#73431,#73432,#73433,#73434,#73435,#73436,#73437,#73438,#73439,#73440,#73441,
#73442,#73443,#73444,#73445,#73446,#73447,#73448,#73449,#73450,#73451,#73452,
#73453,#73454,#73455,#73456,#73457,#73458,#73459,#73460,#73461,#73462,#73463,
#73464,#73465,#73466,#73467,#73468,#73469,#73470,#73471,#73472,#73473,#73474,
#73475,#73476,#73477),.UNSPECIFIED.,.F.,.F.,(4,3,3,3,3,3,3,3,3,3,3,3,3,
3,3,3,3,4),(0.,0.0568525693849193,0.115818688059534,0.173763369030792,0.232053865677185,
0.290632777510717,0.350119962828498,0.409067978904654,0.468824748843247,
0.528581518781839,0.587508828934109,0.646482285375474,0.705424215615768,
0.764242216553829,0.823181662415371,0.881380292059083,0.940690146029541,
1.),.UNSPECIFIED.);
#1627=B_SPLINE_CURVE_WITH_KNOTS('',5,(#73545,#73546,#73547,#73548,#73549,
#73550),.UNSPECIFIED.,.F.,.F.,(6,6),(33.4669635909,40.2517860105),
 .UNSPECIFIED.);
#1628=B_SPLINE_CURVE_WITH_KNOTS('',5,(#73620,#73621,#73622,#73623,#73624,
#73625),.UNSPECIFIED.,.F.,.F.,(6,6),(-1.39421694447,-0.574089330078),
 .UNSPECIFIED.);
#1629=B_SPLINE_CURVE_WITH_KNOTS('',5,(#73733,#73734,#73735,#73736,#73737,
#73738,#73739,#73740,#73741,#73742,#73743,#73744,#73745,#73746,#73747),
 .UNSPECIFIED.,.F.,.F.,(6,3,3,3,6),(-39.7897545658,-32.2822537043,-24.7747528429,
-17.2672519814,-9.75975111992),.UNSPECIFIED.);
#1630=B_SPLINE_CURVE_WITH_KNOTS('',5,(#73835,#73836,#73837,#73838,#73839,
#73840),.UNSPECIFIED.,.F.,.F.,(6,6),(-0.336376155459,0.336376155459),
 .UNSPECIFIED.);
#1631=B_SPLINE_CURVE_WITH_KNOTS('',5,(#73910,#73911,#73912,#73913,#73914,
#73915),.UNSPECIFIED.,.F.,.F.,(6,6),(-0.336376155459,0.336376155459),
 .UNSPECIFIED.);
#1632=B_SPLINE_CURVE_WITH_KNOTS('',5,(#74021,#74022,#74023,#74024,#74025,
#74026,#74027,#74028,#74029,#74030,#74031,#74032,#74033,#74034,#74035),
 .UNSPECIFIED.,.F.,.F.,(6,3,3,3,6),(-39.7897545658,-32.2822537043,-24.7747528429,
-17.2672519814,-9.75975111992),.UNSPECIFIED.);
#1633=B_SPLINE_CURVE_WITH_KNOTS('',5,(#74123,#74124,#74125,#74126,#74127,
#74128),.UNSPECIFIED.,.F.,.F.,(6,6),(-1.39421694447,-0.574089330078),
 .UNSPECIFIED.);
#1634=B_SPLINE_CURVE_WITH_KNOTS('',5,(#74204,#74205,#74206,#74207,#74208,
#74209),.UNSPECIFIED.,.F.,.F.,(6,6),(-4.90357559929,4.90357559929),
 .UNSPECIFIED.);
#1635=B_SPLINE_CURVE_WITH_KNOTS('',5,(#74279,#74280,#74281,#74282,#74283,
#74284),.UNSPECIFIED.,.F.,.F.,(6,6),(-4.90357559929,4.90357559929),
 .UNSPECIFIED.);
#2046=SHAPE_REPRESENTATION_RELATIONSHIP('SRR','None',#98343,#2056);
#2056=ADVANCED_BREP_SHAPE_REPRESENTATION('',(#2076),#98295);
#2066=STYLED_ITEM('',(#98399),#2076);
#2076=MANIFOLD_SOLID_BREP('Body1',#34170);
#2125=PLANE('',#34921);
#2126=PLANE('',#34924);
#2127=PLANE('',#34939);
#2128=PLANE('',#34944);
#2129=PLANE('',#34957);
#2130=PLANE('',#34961);
#2614=CYLINDRICAL_SURFACE('',#34930,5.5);
#2615=CYLINDRICAL_SURFACE('',#34934,5.5);
#2616=CYLINDRICAL_SURFACE('',#34937,0.3);
#2617=CYLINDRICAL_SURFACE('',#34942,0.3);
#2618=CYLINDRICAL_SURFACE('',#34955,0.3);
#2619=CYLINDRICAL_SURFACE('',#34960,0.3);
#3685=FACE_OUTER_BOUND('',#5839,.T.);
#3686=FACE_OUTER_BOUND('',#5843,.T.);
#3687=FACE_OUTER_BOUND('',#5847,.T.);
#3688=FACE_OUTER_BOUND('',#5848,.T.);
#3689=FACE_OUTER_BOUND('',#5849,.T.);
#3690=FACE_OUTER_BOUND('',#5850,.T.);
#3691=FACE_OUTER_BOUND('',#5851,.T.);
#3692=FACE_OUTER_BOUND('',#5852,.T.);
#3693=FACE_OUTER_BOUND('',#5853,.T.);
#3694=FACE_OUTER_BOUND('',#5854,.T.);
#3695=FACE_OUTER_BOUND('',#5855,.T.);
#3696=FACE_OUTER_BOUND('',#5856,.T.);
#3697=FACE_OUTER_BOUND('',#5857,.T.);
#3698=FACE_OUTER_BOUND('',#5858,.T.);
#3699=FACE_OUTER_BOUND('',#5859,.T.);
#3700=FACE_OUTER_BOUND('',#5860,.T.);
#3701=FACE_OUTER_BOUND('',#5861,.T.);
#3702=FACE_OUTER_BOUND('',#5862,.T.);
#3703=FACE_OUTER_BOUND('',#5863,.T.);
#3704=FACE_OUTER_BOUND('',#5864,.T.);
#3705=FACE_OUTER_BOUND('',#5865,.T.);
#3706=FACE_OUTER_BOUND('',#5866,.T.);
#3707=FACE_OUTER_BOUND('',#5867,.T.);
#3708=FACE_OUTER_BOUND('',#5868,.T.);
#3709=FACE_OUTER_BOUND('',#5869,.T.);
#3710=FACE_OUTER_BOUND('',#5870,.T.);
#3711=FACE_OUTER_BOUND('',#5871,.T.);
#3712=FACE_OUTER_BOUND('',#5872,.T.);
#3713=FACE_OUTER_BOUND('',#5873,.T.);
#3714=FACE_OUTER_BOUND('',#5874,.T.);
#3715=FACE_OUTER_BOUND('',#5875,.T.);
#3716=FACE_OUTER_BOUND('',#5876,.T.);
#3717=FACE_OUTER_BOUND('',#5877,.T.);
#3718=FACE_OUTER_BOUND('',#5878,.T.);
#3719=FACE_OUTER_BOUND('',#5879,.T.);
#3720=FACE_OUTER_BOUND('',#5880,.T.);
#3721=FACE_OUTER_BOUND('',#5881,.T.);
#3722=FACE_OUTER_BOUND('',#5882,.T.);
#3723=FACE_OUTER_BOUND('',#5883,.T.);
#3724=FACE_OUTER_BOUND('',#5884,.T.);
#3725=FACE_OUTER_BOUND('',#5885,.T.);
#3726=FACE_OUTER_BOUND('',#5886,.T.);
#3727=FACE_OUTER_BOUND('',#5887,.T.);
#3728=FACE_OUTER_BOUND('',#5888,.T.);
#5839=EDGE_LOOP('',(#23727,#23728,#23729,#23730,#23731,#23732,#23733,#23734,
#23735,#23736));
#5840=EDGE_LOOP('',(#23737,#23738,#23739,#23740,#23741,#23742,#23743,#23744,
#23745));
#5841=EDGE_LOOP('',(#23746));
#5842=EDGE_LOOP('',(#23747));
#5843=EDGE_LOOP('',(#23748,#23749,#23750,#23751,#23752,#23753,#23754,#23755,
#23756,#23757));
#5844=EDGE_LOOP('',(#23758));
#5845=EDGE_LOOP('',(#23759));
#5846=EDGE_LOOP('',(#23760,#23761,#23762,#23763,#23764,#23765,#23766,#23767,
#23768));
#5847=EDGE_LOOP('',(#23769,#23770,#23771,#23772));
#5848=EDGE_LOOP('',(#23773,#23774,#23775,#23776));
#5849=EDGE_LOOP('',(#23777,#23778,#23779,#23780));
#5850=EDGE_LOOP('',(#23781,#23782,#23783,#23784));
#5851=EDGE_LOOP('',(#23785,#23786,#23787,#23788));
#5852=EDGE_LOOP('',(#23789,#23790,#23791,#23792));
#5853=EDGE_LOOP('',(#23793,#23794,#23795,#23796));
#5854=EDGE_LOOP('',(#23797,#23798,#23799,#23800));
#5855=EDGE_LOOP('',(#23801,#23802,#23803,#23804));
#5856=EDGE_LOOP('',(#23805,#23806,#23807,#23808));
#5857=EDGE_LOOP('',(#23809,#23810,#23811,#23812));
#5858=EDGE_LOOP('',(#23813,#23814,#23815,#23816));
#5859=EDGE_LOOP('',(#23817,#23818,#23819,#23820));
#5860=EDGE_LOOP('',(#23821,#23822,#23823,#23824));
#5861=EDGE_LOOP('',(#23825,#23826,#23827,#23828));
#5862=EDGE_LOOP('',(#23829,#23830,#23831,#23832));
#5863=EDGE_LOOP('',(#23833,#23834,#23835,#23836));
#5864=EDGE_LOOP('',(#23837,#23838,#23839,#23840));
#5865=EDGE_LOOP('',(#23841,#23842,#23843,#23844));
#5866=EDGE_LOOP('',(#23845,#23846,#23847,#23848));
#5867=EDGE_LOOP('',(#23849,#23850,#23851,#23852));
#5868=EDGE_LOOP('',(#23853,#23854,#23855,#23856));
#5869=EDGE_LOOP('',(#23857,#23858,#23859,#23860));
#5870=EDGE_LOOP('',(#23861,#23862,#23863,#23864));
#5871=EDGE_LOOP('',(#23865,#23866,#23867,#23868));
#5872=EDGE_LOOP('',(#23869,#23870,#23871,#23872));
#5873=EDGE_LOOP('',(#23873,#23874,#23875,#23876));
#5874=EDGE_LOOP('',(#23877,#23878,#23879,#23880));
#5875=EDGE_LOOP('',(#23881,#23882,#23883,#23884));
#5876=EDGE_LOOP('',(#23885,#23886,#23887,#23888));
#5877=EDGE_LOOP('',(#23889,#23890,#23891,#23892));
#5878=EDGE_LOOP('',(#23893,#23894,#23895,#23896));
#5879=EDGE_LOOP('',(#23897,#23898,#23899,#23900));
#5880=EDGE_LOOP('',(#23901,#23902,#23903,#23904));
#5881=EDGE_LOOP('',(#23905,#23906,#23907,#23908));
#5882=EDGE_LOOP('',(#23909,#23910,#23911,#23912));
#5883=EDGE_LOOP('',(#23913,#23914,#23915,#23916));
#5884=EDGE_LOOP('',(#23917,#23918,#23919,#23920));
#5885=EDGE_LOOP('',(#23921,#23922,#23923,#23924));
#5886=EDGE_LOOP('',(#23925,#23926,#23927,#23928));
#5887=EDGE_LOOP('',(#23929,#23930,#23931,#23932));
#5888=EDGE_LOOP('',(#23933,#23934,#23935,#23936));
#7916=LINE('',#71967,#9756);
#7917=LINE('',#72093,#9757);
#7918=LINE('',#72397,#9758);
#7919=LINE('',#72646,#9759);
#7920=LINE('',#72843,#9760);
#7921=LINE('',#72858,#9761);
#7922=LINE('',#72872,#9762);
#7923=LINE('',#72888,#9763);
#7924=LINE('',#72921,#9764);
#7925=LINE('',#72927,#9765);
#7926=LINE('',#73004,#9766);
#7927=LINE('',#73005,#9767);
#7928=LINE('',#73009,#9768);
#7929=LINE('',#73011,#9769);
#7930=LINE('',#73086,#9770);
#7931=LINE('',#73213,#9771);
#7932=LINE('',#73217,#9772);
#7933=LINE('',#73219,#9773);
#7934=LINE('',#73294,#9774);
#7935=LINE('',#73369,#9775);
#7936=LINE('',#73490,#9776);
#7937=LINE('',#73639,#9777);
#7938=LINE('',#73640,#9778);
#7939=LINE('',#73778,#9779);
#7940=LINE('',#73853,#9780);
#7941=LINE('',#73928,#9781);
#7942=LINE('',#74066,#9782);
#7943=LINE('',#74141,#9783);
#7944=LINE('',#74145,#9784);
#7945=LINE('',#74147,#9785);
#7946=LINE('',#74222,#9786);
#7947=LINE('',#74297,#9787);
#7948=LINE('',#74299,#9788);
#9756=VECTOR('',#40159,1000.);
#9757=VECTOR('',#40160,1000.);
#9758=VECTOR('',#40161,1000.);
#9759=VECTOR('',#40162,1000.);
#9760=VECTOR('',#40169,1000.);
#9761=VECTOR('',#40170,1000.);
#9762=VECTOR('',#40175,1000.);
#9763=VECTOR('',#40176,1000.);
#9764=VECTOR('',#40185,5.5);
#9765=VECTOR('',#40194,5.5);
#9766=VECTOR('',#40199,1000.);
#9767=VECTOR('',#40200,1000.);
#9768=VECTOR('',#40205,1000.);
#9769=VECTOR('',#40208,1000.);
#9770=VECTOR('',#40211,1000.);
#9771=VECTOR('',#40214,1000.);
#9772=VECTOR('',#40219,1000.);
#9773=VECTOR('',#40222,1000.);
#9774=VECTOR('',#40225,1000.);
#9775=VECTOR('',#40228,1000.);
#9776=VECTOR('',#40231,1000.);
#9777=VECTOR('',#40236,1000.);
#9778=VECTOR('',#40237,1000.);
#9779=VECTOR('',#40240,1000.);
#9780=VECTOR('',#40243,1000.);
#9781=VECTOR('',#40246,1000.);
#9782=VECTOR('',#40249,1000.);
#9783=VECTOR('',#40252,1000.);
#9784=VECTOR('',#40257,1000.);
#9785=VECTOR('',#40260,1000.);
#9786=VECTOR('',#40263,1000.);
#9787=VECTOR('',#40266,1000.);
#9788=VECTOR('',#40269,1000.);
#11631=CIRCLE('',#34922,5.8);
#11632=CIRCLE('',#34923,5.8);
#11633=CIRCLE('',#34925,5.5);
#11634=CIRCLE('',#34926,5.5);
#11635=CIRCLE('',#34928,5.5);
#11636=CIRCLE('',#34929,0.3);
#11637=CIRCLE('',#34932,5.5);
#11638=CIRCLE('',#34933,0.3);
#11639=CIRCLE('',#34938,0.300000000000002);
#14199=VERTEX_POINT('',#71742);
#14200=VERTEX_POINT('',#71743);
#14201=VERTEX_POINT('',#71919);
#14202=VERTEX_POINT('',#71966);
#14203=VERTEX_POINT('',#71968);
#14204=VERTEX_POINT('',#72030);
#14205=VERTEX_POINT('',#72092);
#14206=VERTEX_POINT('',#72094);
#14207=VERTEX_POINT('',#72141);
#14208=VERTEX_POINT('',#72314);
#14209=VERTEX_POINT('',#72395);
#14210=VERTEX_POINT('',#72396);
#14211=VERTEX_POINT('',#72398);
#14212=VERTEX_POINT('',#72439);
#14213=VERTEX_POINT('',#72483);
#14214=VERTEX_POINT('',#72560);
#14215=VERTEX_POINT('',#72607);
#14216=VERTEX_POINT('',#72645);
#14217=VERTEX_POINT('',#72647);
#14218=VERTEX_POINT('',#72776);
#14219=VERTEX_POINT('',#72778);
#14220=VERTEX_POINT('',#72781);
#14221=VERTEX_POINT('',#72782);
#14222=VERTEX_POINT('',#72789);
#14223=VERTEX_POINT('',#72805);
#14224=VERTEX_POINT('',#72812);
#14225=VERTEX_POINT('',#72819);
#14226=VERTEX_POINT('',#72835);
#14227=VERTEX_POINT('',#72842);
#14228=VERTEX_POINT('',#72844);
#14229=VERTEX_POINT('',#72851);
#14230=VERTEX_POINT('',#72859);
#14231=VERTEX_POINT('',#72861);
#14232=VERTEX_POINT('',#72863);
#14233=VERTEX_POINT('',#72864);
#14234=VERTEX_POINT('',#72871);
#14235=VERTEX_POINT('',#72873);
#14236=VERTEX_POINT('',#72880);
#14237=VERTEX_POINT('',#72887);
#14238=VERTEX_POINT('',#72889);
#14239=VERTEX_POINT('',#72896);
#14240=VERTEX_POINT('',#72903);
#14241=VERTEX_POINT('',#72917);
#14242=VERTEX_POINT('',#72923);
#14243=VERTEX_POINT('',#72982);
#14244=VERTEX_POINT('',#72984);
#14245=VERTEX_POINT('',#73007);
#14246=VERTEX_POINT('',#73066);
#14247=VERTEX_POINT('',#73141);
#14248=VERTEX_POINT('',#73215);
#14249=VERTEX_POINT('',#73274);
#14250=VERTEX_POINT('',#73349);
#14251=VERTEX_POINT('',#73424);
#14252=VERTEX_POINT('',#73617);
#14253=VERTEX_POINT('',#73619);
#14254=VERTEX_POINT('',#73731);
#14255=VERTEX_POINT('',#73833);
#14256=VERTEX_POINT('',#73908);
#14257=VERTEX_POINT('',#74019);
#14258=VERTEX_POINT('',#74121);
#14259=VERTEX_POINT('',#74143);
#14260=VERTEX_POINT('',#74202);
#14261=VERTEX_POINT('',#74277);
#17635=EDGE_CURVE('',#14199,#14200,#1591,.T.);
#17636=EDGE_CURVE('',#14200,#14201,#1592,.T.);
#17637=EDGE_CURVE('',#14201,#14202,#7916,.T.);
#17638=EDGE_CURVE('',#14202,#14203,#1593,.T.);
#17639=EDGE_CURVE('',#14203,#14204,#1594,.T.);
#17640=EDGE_CURVE('',#14204,#14205,#7917,.T.);
#17641=EDGE_CURVE('',#14205,#14206,#1595,.T.);
#17642=EDGE_CURVE('',#14206,#14207,#1596,.T.);
#17643=EDGE_CURVE('',#14207,#14208,#1597,.T.);
#17644=EDGE_CURVE('',#14208,#14199,#1598,.T.);
#17645=EDGE_CURVE('',#14209,#14210,#7918,.T.);
#17646=EDGE_CURVE('',#14211,#14209,#1599,.T.);
#17647=EDGE_CURVE('',#14212,#14211,#1600,.T.);
#17648=EDGE_CURVE('',#14213,#14212,#1601,.T.);
#17649=EDGE_CURVE('',#14214,#14213,#1602,.T.);
#17650=EDGE_CURVE('',#14215,#14214,#1603,.T.);
#17651=EDGE_CURVE('',#14216,#14215,#7919,.T.);
#17652=EDGE_CURVE('',#14217,#14216,#1604,.T.);
#17653=EDGE_CURVE('',#14210,#14217,#1605,.T.);
#17654=EDGE_CURVE('',#14218,#14218,#11631,.T.);
#17655=EDGE_CURVE('',#14219,#14219,#11632,.T.);
#17656=EDGE_CURVE('',#14220,#14221,#1606,.T.);
#17657=EDGE_CURVE('',#14222,#14220,#1607,.T.);
#17658=EDGE_CURVE('',#14223,#14222,#1608,.T.);
#17659=EDGE_CURVE('',#14224,#14223,#1609,.T.);
#17660=EDGE_CURVE('',#14225,#14224,#1610,.T.);
#17661=EDGE_CURVE('',#14226,#14225,#1611,.T.);
#17662=EDGE_CURVE('',#14227,#14226,#7920,.T.);
#17663=EDGE_CURVE('',#14228,#14227,#1612,.T.);
#17664=EDGE_CURVE('',#14229,#14228,#1613,.T.);
#17665=EDGE_CURVE('',#14221,#14229,#7921,.T.);
#17666=EDGE_CURVE('',#14230,#14230,#11633,.T.);
#17667=EDGE_CURVE('',#14231,#14231,#11634,.T.);
#17668=EDGE_CURVE('',#14232,#14233,#1614,.T.);
#17669=EDGE_CURVE('',#14233,#14234,#7922,.T.);
#17670=EDGE_CURVE('',#14234,#14235,#1615,.T.);
#17671=EDGE_CURVE('',#14235,#14236,#1616,.T.);
#17672=EDGE_CURVE('',#14236,#14237,#7923,.T.);
#17673=EDGE_CURVE('',#14237,#14238,#1617,.T.);
#17674=EDGE_CURVE('',#14238,#14239,#1618,.T.);
#17675=EDGE_CURVE('',#14239,#14240,#1619,.T.);
#17676=EDGE_CURVE('',#14240,#14232,#1620,.T.);
#17677=EDGE_CURVE('',#14241,#14241,#11635,.T.);
#17678=EDGE_CURVE('',#14241,#14219,#11636,.T.);
#17679=EDGE_CURVE('',#14230,#14241,#7924,.T.);
#17680=EDGE_CURVE('',#14242,#14242,#11637,.T.);
#17681=EDGE_CURVE('',#14242,#14218,#11638,.T.);
#17682=EDGE_CURVE('',#14231,#14242,#7925,.T.);
#17683=EDGE_CURVE('',#14243,#14211,#569,.T.);
#17684=EDGE_CURVE('',#14244,#14209,#570,.T.);
#17685=EDGE_CURVE('',#14243,#14244,#1621,.T.);
#17686=EDGE_CURVE('',#14233,#14244,#7926,.T.);
#17687=EDGE_CURVE('',#14232,#14243,#7927,.T.);
#17688=EDGE_CURVE('',#14245,#14210,#11639,.T.);
#17689=EDGE_CURVE('',#14244,#14245,#7928,.T.);
#17690=EDGE_CURVE('',#14234,#14245,#7929,.T.);
#17691=EDGE_CURVE('',#14246,#14217,#571,.T.);
#17692=EDGE_CURVE('',#14245,#14246,#1622,.T.);
#17693=EDGE_CURVE('',#14235,#14246,#7930,.T.);
#17694=EDGE_CURVE('',#14247,#14216,#572,.T.);
#17695=EDGE_CURVE('',#14246,#14247,#1623,.T.);
#17696=EDGE_CURVE('',#14236,#14247,#7931,.T.);
#17697=EDGE_CURVE('',#14248,#14215,#573,.T.);
#17698=EDGE_CURVE('',#14247,#14248,#7932,.T.);
#17699=EDGE_CURVE('',#14237,#14248,#7933,.T.);
#17700=EDGE_CURVE('',#14249,#14214,#574,.T.);
#17701=EDGE_CURVE('',#14248,#14249,#1624,.T.);
#17702=EDGE_CURVE('',#14238,#14249,#7934,.T.);
#17703=EDGE_CURVE('',#14250,#14213,#575,.T.);
#17704=EDGE_CURVE('',#14249,#14250,#1625,.T.);
#17705=EDGE_CURVE('',#14239,#14250,#7935,.T.);
#17706=EDGE_CURVE('',#14251,#14212,#576,.T.);
#17707=EDGE_CURVE('',#14250,#14251,#1626,.T.);
#17708=EDGE_CURVE('',#14240,#14251,#7936,.T.);
#17709=EDGE_CURVE('',#14251,#14243,#1627,.T.);
#17710=EDGE_CURVE('',#14200,#14252,#577,.T.);
#17711=EDGE_CURVE('',#14252,#14253,#1628,.T.);
#17712=EDGE_CURVE('',#14201,#14253,#578,.T.);
#17713=EDGE_CURVE('',#14220,#14252,#7937,.T.);
#17714=EDGE_CURVE('',#14221,#14253,#7938,.T.);
#17715=EDGE_CURVE('',#14199,#14254,#579,.T.);
#17716=EDGE_CURVE('',#14254,#14252,#1629,.T.);
#17717=EDGE_CURVE('',#14222,#14254,#7939,.T.);
#17718=EDGE_CURVE('',#14208,#14255,#580,.T.);
#17719=EDGE_CURVE('',#14255,#14254,#1630,.T.);
#17720=EDGE_CURVE('',#14223,#14255,#7940,.T.);
#17721=EDGE_CURVE('',#14207,#14256,#581,.T.);
#17722=EDGE_CURVE('',#14256,#14255,#1631,.T.);
#17723=EDGE_CURVE('',#14224,#14256,#7941,.T.);
#17724=EDGE_CURVE('',#14206,#14257,#582,.T.);
#17725=EDGE_CURVE('',#14257,#14256,#1632,.T.);
#17726=EDGE_CURVE('',#14225,#14257,#7942,.T.);
#17727=EDGE_CURVE('',#14205,#14258,#583,.T.);
#17728=EDGE_CURVE('',#14258,#14257,#1633,.T.);
#17729=EDGE_CURVE('',#14226,#14258,#7943,.T.);
#17730=EDGE_CURVE('',#14204,#14259,#584,.T.);
#17731=EDGE_CURVE('',#14259,#14258,#7944,.T.);
#17732=EDGE_CURVE('',#14227,#14259,#7945,.T.);
#17733=EDGE_CURVE('',#14203,#14260,#585,.T.);
#17734=EDGE_CURVE('',#14260,#14259,#1634,.T.);
#17735=EDGE_CURVE('',#14228,#14260,#7946,.T.);
#17736=EDGE_CURVE('',#14202,#14261,#586,.T.);
#17737=EDGE_CURVE('',#14261,#14260,#1635,.T.);
#17738=EDGE_CURVE('',#14229,#14261,#7947,.T.);
#17739=EDGE_CURVE('',#14253,#14261,#7948,.T.);
#23727=ORIENTED_EDGE('',*,*,#17635,.T.);
#23728=ORIENTED_EDGE('',*,*,#17636,.T.);
#23729=ORIENTED_EDGE('',*,*,#17637,.T.);
#23730=ORIENTED_EDGE('',*,*,#17638,.T.);
#23731=ORIENTED_EDGE('',*,*,#17639,.T.);
#23732=ORIENTED_EDGE('',*,*,#17640,.T.);
#23733=ORIENTED_EDGE('',*,*,#17641,.T.);
#23734=ORIENTED_EDGE('',*,*,#17642,.T.);
#23735=ORIENTED_EDGE('',*,*,#17643,.T.);
#23736=ORIENTED_EDGE('',*,*,#17644,.T.);
#23737=ORIENTED_EDGE('',*,*,#17645,.F.);
#23738=ORIENTED_EDGE('',*,*,#17646,.F.);
#23739=ORIENTED_EDGE('',*,*,#17647,.F.);
#23740=ORIENTED_EDGE('',*,*,#17648,.F.);
#23741=ORIENTED_EDGE('',*,*,#17649,.F.);
#23742=ORIENTED_EDGE('',*,*,#17650,.F.);
#23743=ORIENTED_EDGE('',*,*,#17651,.F.);
#23744=ORIENTED_EDGE('',*,*,#17652,.F.);
#23745=ORIENTED_EDGE('',*,*,#17653,.F.);
#23746=ORIENTED_EDGE('',*,*,#17654,.F.);
#23747=ORIENTED_EDGE('',*,*,#17655,.F.);
#23748=ORIENTED_EDGE('',*,*,#17656,.F.);
#23749=ORIENTED_EDGE('',*,*,#17657,.F.);
#23750=ORIENTED_EDGE('',*,*,#17658,.F.);
#23751=ORIENTED_EDGE('',*,*,#17659,.F.);
#23752=ORIENTED_EDGE('',*,*,#17660,.F.);
#23753=ORIENTED_EDGE('',*,*,#17661,.F.);
#23754=ORIENTED_EDGE('',*,*,#17662,.F.);
#23755=ORIENTED_EDGE('',*,*,#17663,.F.);
#23756=ORIENTED_EDGE('',*,*,#17664,.F.);
#23757=ORIENTED_EDGE('',*,*,#17665,.F.);
#23758=ORIENTED_EDGE('',*,*,#17666,.T.);
#23759=ORIENTED_EDGE('',*,*,#17667,.T.);
#23760=ORIENTED_EDGE('',*,*,#17668,.T.);
#23761=ORIENTED_EDGE('',*,*,#17669,.T.);
#23762=ORIENTED_EDGE('',*,*,#17670,.T.);
#23763=ORIENTED_EDGE('',*,*,#17671,.T.);
#23764=ORIENTED_EDGE('',*,*,#17672,.T.);
#23765=ORIENTED_EDGE('',*,*,#17673,.T.);
#23766=ORIENTED_EDGE('',*,*,#17674,.T.);
#23767=ORIENTED_EDGE('',*,*,#17675,.T.);
#23768=ORIENTED_EDGE('',*,*,#17676,.T.);
#23769=ORIENTED_EDGE('',*,*,#17677,.F.);
#23770=ORIENTED_EDGE('',*,*,#17678,.T.);
#23771=ORIENTED_EDGE('',*,*,#17655,.T.);
#23772=ORIENTED_EDGE('',*,*,#17678,.F.);
#23773=ORIENTED_EDGE('',*,*,#17666,.F.);
#23774=ORIENTED_EDGE('',*,*,#17679,.T.);
#23775=ORIENTED_EDGE('',*,*,#17677,.T.);
#23776=ORIENTED_EDGE('',*,*,#17679,.F.);
#23777=ORIENTED_EDGE('',*,*,#17680,.F.);
#23778=ORIENTED_EDGE('',*,*,#17681,.T.);
#23779=ORIENTED_EDGE('',*,*,#17654,.T.);
#23780=ORIENTED_EDGE('',*,*,#17681,.F.);
#23781=ORIENTED_EDGE('',*,*,#17667,.F.);
#23782=ORIENTED_EDGE('',*,*,#17682,.T.);
#23783=ORIENTED_EDGE('',*,*,#17680,.T.);
#23784=ORIENTED_EDGE('',*,*,#17682,.F.);
#23785=ORIENTED_EDGE('',*,*,#17683,.T.);
#23786=ORIENTED_EDGE('',*,*,#17646,.T.);
#23787=ORIENTED_EDGE('',*,*,#17684,.F.);
#23788=ORIENTED_EDGE('',*,*,#17685,.F.);
#23789=ORIENTED_EDGE('',*,*,#17685,.T.);
#23790=ORIENTED_EDGE('',*,*,#17686,.F.);
#23791=ORIENTED_EDGE('',*,*,#17668,.F.);
#23792=ORIENTED_EDGE('',*,*,#17687,.T.);
#23793=ORIENTED_EDGE('',*,*,#17684,.T.);
#23794=ORIENTED_EDGE('',*,*,#17645,.T.);
#23795=ORIENTED_EDGE('',*,*,#17688,.F.);
#23796=ORIENTED_EDGE('',*,*,#17689,.F.);
#23797=ORIENTED_EDGE('',*,*,#17689,.T.);
#23798=ORIENTED_EDGE('',*,*,#17690,.F.);
#23799=ORIENTED_EDGE('',*,*,#17669,.F.);
#23800=ORIENTED_EDGE('',*,*,#17686,.T.);
#23801=ORIENTED_EDGE('',*,*,#17688,.T.);
#23802=ORIENTED_EDGE('',*,*,#17653,.T.);
#23803=ORIENTED_EDGE('',*,*,#17691,.F.);
#23804=ORIENTED_EDGE('',*,*,#17692,.F.);
#23805=ORIENTED_EDGE('',*,*,#17692,.T.);
#23806=ORIENTED_EDGE('',*,*,#17693,.F.);
#23807=ORIENTED_EDGE('',*,*,#17670,.F.);
#23808=ORIENTED_EDGE('',*,*,#17690,.T.);
#23809=ORIENTED_EDGE('',*,*,#17691,.T.);
#23810=ORIENTED_EDGE('',*,*,#17652,.T.);
#23811=ORIENTED_EDGE('',*,*,#17694,.F.);
#23812=ORIENTED_EDGE('',*,*,#17695,.F.);
#23813=ORIENTED_EDGE('',*,*,#17695,.T.);
#23814=ORIENTED_EDGE('',*,*,#17696,.F.);
#23815=ORIENTED_EDGE('',*,*,#17671,.F.);
#23816=ORIENTED_EDGE('',*,*,#17693,.T.);
#23817=ORIENTED_EDGE('',*,*,#17694,.T.);
#23818=ORIENTED_EDGE('',*,*,#17651,.T.);
#23819=ORIENTED_EDGE('',*,*,#17697,.F.);
#23820=ORIENTED_EDGE('',*,*,#17698,.F.);
#23821=ORIENTED_EDGE('',*,*,#17698,.T.);
#23822=ORIENTED_EDGE('',*,*,#17699,.F.);
#23823=ORIENTED_EDGE('',*,*,#17672,.F.);
#23824=ORIENTED_EDGE('',*,*,#17696,.T.);
#23825=ORIENTED_EDGE('',*,*,#17697,.T.);
#23826=ORIENTED_EDGE('',*,*,#17650,.T.);
#23827=ORIENTED_EDGE('',*,*,#17700,.F.);
#23828=ORIENTED_EDGE('',*,*,#17701,.F.);
#23829=ORIENTED_EDGE('',*,*,#17701,.T.);
#23830=ORIENTED_EDGE('',*,*,#17702,.F.);
#23831=ORIENTED_EDGE('',*,*,#17673,.F.);
#23832=ORIENTED_EDGE('',*,*,#17699,.T.);
#23833=ORIENTED_EDGE('',*,*,#17700,.T.);
#23834=ORIENTED_EDGE('',*,*,#17649,.T.);
#23835=ORIENTED_EDGE('',*,*,#17703,.F.);
#23836=ORIENTED_EDGE('',*,*,#17704,.F.);
#23837=ORIENTED_EDGE('',*,*,#17704,.T.);
#23838=ORIENTED_EDGE('',*,*,#17705,.F.);
#23839=ORIENTED_EDGE('',*,*,#17674,.F.);
#23840=ORIENTED_EDGE('',*,*,#17702,.T.);
#23841=ORIENTED_EDGE('',*,*,#17703,.T.);
#23842=ORIENTED_EDGE('',*,*,#17648,.T.);
#23843=ORIENTED_EDGE('',*,*,#17706,.F.);
#23844=ORIENTED_EDGE('',*,*,#17707,.F.);
#23845=ORIENTED_EDGE('',*,*,#17707,.T.);
#23846=ORIENTED_EDGE('',*,*,#17708,.F.);
#23847=ORIENTED_EDGE('',*,*,#17675,.F.);
#23848=ORIENTED_EDGE('',*,*,#17705,.T.);
#23849=ORIENTED_EDGE('',*,*,#17706,.T.);
#23850=ORIENTED_EDGE('',*,*,#17647,.T.);
#23851=ORIENTED_EDGE('',*,*,#17683,.F.);
#23852=ORIENTED_EDGE('',*,*,#17709,.F.);
#23853=ORIENTED_EDGE('',*,*,#17709,.T.);
#23854=ORIENTED_EDGE('',*,*,#17687,.F.);
#23855=ORIENTED_EDGE('',*,*,#17676,.F.);
#23856=ORIENTED_EDGE('',*,*,#17708,.T.);
#23857=ORIENTED_EDGE('',*,*,#17710,.T.);
#23858=ORIENTED_EDGE('',*,*,#17711,.T.);
#23859=ORIENTED_EDGE('',*,*,#17712,.F.);
#23860=ORIENTED_EDGE('',*,*,#17636,.F.);
#23861=ORIENTED_EDGE('',*,*,#17711,.F.);
#23862=ORIENTED_EDGE('',*,*,#17713,.F.);
#23863=ORIENTED_EDGE('',*,*,#17656,.T.);
#23864=ORIENTED_EDGE('',*,*,#17714,.T.);
#23865=ORIENTED_EDGE('',*,*,#17715,.T.);
#23866=ORIENTED_EDGE('',*,*,#17716,.T.);
#23867=ORIENTED_EDGE('',*,*,#17710,.F.);
#23868=ORIENTED_EDGE('',*,*,#17635,.F.);
#23869=ORIENTED_EDGE('',*,*,#17716,.F.);
#23870=ORIENTED_EDGE('',*,*,#17717,.F.);
#23871=ORIENTED_EDGE('',*,*,#17657,.T.);
#23872=ORIENTED_EDGE('',*,*,#17713,.T.);
#23873=ORIENTED_EDGE('',*,*,#17718,.T.);
#23874=ORIENTED_EDGE('',*,*,#17719,.T.);
#23875=ORIENTED_EDGE('',*,*,#17715,.F.);
#23876=ORIENTED_EDGE('',*,*,#17644,.F.);
#23877=ORIENTED_EDGE('',*,*,#17719,.F.);
#23878=ORIENTED_EDGE('',*,*,#17720,.F.);
#23879=ORIENTED_EDGE('',*,*,#17658,.T.);
#23880=ORIENTED_EDGE('',*,*,#17717,.T.);
#23881=ORIENTED_EDGE('',*,*,#17721,.T.);
#23882=ORIENTED_EDGE('',*,*,#17722,.T.);
#23883=ORIENTED_EDGE('',*,*,#17718,.F.);
#23884=ORIENTED_EDGE('',*,*,#17643,.F.);
#23885=ORIENTED_EDGE('',*,*,#17722,.F.);
#23886=ORIENTED_EDGE('',*,*,#17723,.F.);
#23887=ORIENTED_EDGE('',*,*,#17659,.T.);
#23888=ORIENTED_EDGE('',*,*,#17720,.T.);
#23889=ORIENTED_EDGE('',*,*,#17724,.T.);
#23890=ORIENTED_EDGE('',*,*,#17725,.T.);
#23891=ORIENTED_EDGE('',*,*,#17721,.F.);
#23892=ORIENTED_EDGE('',*,*,#17642,.F.);
#23893=ORIENTED_EDGE('',*,*,#17725,.F.);
#23894=ORIENTED_EDGE('',*,*,#17726,.F.);
#23895=ORIENTED_EDGE('',*,*,#17660,.T.);
#23896=ORIENTED_EDGE('',*,*,#17723,.T.);
#23897=ORIENTED_EDGE('',*,*,#17727,.T.);
#23898=ORIENTED_EDGE('',*,*,#17728,.T.);
#23899=ORIENTED_EDGE('',*,*,#17724,.F.);
#23900=ORIENTED_EDGE('',*,*,#17641,.F.);
#23901=ORIENTED_EDGE('',*,*,#17728,.F.);
#23902=ORIENTED_EDGE('',*,*,#17729,.F.);
#23903=ORIENTED_EDGE('',*,*,#17661,.T.);
#23904=ORIENTED_EDGE('',*,*,#17726,.T.);
#23905=ORIENTED_EDGE('',*,*,#17730,.T.);
#23906=ORIENTED_EDGE('',*,*,#17731,.T.);
#23907=ORIENTED_EDGE('',*,*,#17727,.F.);
#23908=ORIENTED_EDGE('',*,*,#17640,.F.);
#23909=ORIENTED_EDGE('',*,*,#17731,.F.);
#23910=ORIENTED_EDGE('',*,*,#17732,.F.);
#23911=ORIENTED_EDGE('',*,*,#17662,.T.);
#23912=ORIENTED_EDGE('',*,*,#17729,.T.);
#23913=ORIENTED_EDGE('',*,*,#17733,.T.);
#23914=ORIENTED_EDGE('',*,*,#17734,.T.);
#23915=ORIENTED_EDGE('',*,*,#17730,.F.);
#23916=ORIENTED_EDGE('',*,*,#17639,.F.);
#23917=ORIENTED_EDGE('',*,*,#17734,.F.);
#23918=ORIENTED_EDGE('',*,*,#17735,.F.);
#23919=ORIENTED_EDGE('',*,*,#17663,.T.);
#23920=ORIENTED_EDGE('',*,*,#17732,.T.);
#23921=ORIENTED_EDGE('',*,*,#17736,.T.);
#23922=ORIENTED_EDGE('',*,*,#17737,.T.);
#23923=ORIENTED_EDGE('',*,*,#17733,.F.);
#23924=ORIENTED_EDGE('',*,*,#17638,.F.);
#23925=ORIENTED_EDGE('',*,*,#17737,.F.);
#23926=ORIENTED_EDGE('',*,*,#17738,.F.);
#23927=ORIENTED_EDGE('',*,*,#17664,.T.);
#23928=ORIENTED_EDGE('',*,*,#17735,.T.);
#23929=ORIENTED_EDGE('',*,*,#17712,.T.);
#23930=ORIENTED_EDGE('',*,*,#17739,.T.);
#23931=ORIENTED_EDGE('',*,*,#17736,.F.);
#23932=ORIENTED_EDGE('',*,*,#17637,.F.);
#23933=ORIENTED_EDGE('',*,*,#17739,.F.);
#23934=ORIENTED_EDGE('',*,*,#17714,.F.);
#23935=ORIENTED_EDGE('',*,*,#17665,.T.);
#23936=ORIENTED_EDGE('',*,*,#17738,.T.);
#32433=ADVANCED_FACE('',(#3685,#1268,#1269,#1270),#2125,.T.);
#32434=ADVANCED_FACE('',(#3686,#1271,#1272,#1273),#2126,.F.);
#32435=ADVANCED_FACE('',(#3687),#118,.T.);
#32436=ADVANCED_FACE('',(#3688),#2614,.F.);
#32437=ADVANCED_FACE('',(#3689),#119,.T.);
#32438=ADVANCED_FACE('',(#3690),#2615,.F.);
#32439=ADVANCED_FACE('',(#3691),#1076,.T.);
#32440=ADVANCED_FACE('',(#3692),#1077,.F.);
#32441=ADVANCED_FACE('',(#3693),#2616,.T.);
#32442=ADVANCED_FACE('',(#3694),#2127,.F.);
#32443=ADVANCED_FACE('',(#3695),#1078,.T.);
#32444=ADVANCED_FACE('',(#3696),#1079,.F.);
#32445=ADVANCED_FACE('',(#3697),#1080,.T.);
#32446=ADVANCED_FACE('',(#3698),#1081,.F.);
#32447=ADVANCED_FACE('',(#3699),#2617,.T.);
#32448=ADVANCED_FACE('',(#3700),#2128,.F.);
#32449=ADVANCED_FACE('',(#3701),#1082,.T.);
#32450=ADVANCED_FACE('',(#3702),#1083,.F.);
#32451=ADVANCED_FACE('',(#3703),#1084,.T.);
#32452=ADVANCED_FACE('',(#3704),#1085,.F.);
#32453=ADVANCED_FACE('',(#3705),#1086,.T.);
#32454=ADVANCED_FACE('',(#3706),#1087,.F.);
#32455=ADVANCED_FACE('',(#3707),#1088,.T.);
#32456=ADVANCED_FACE('',(#3708),#1089,.F.);
#32457=ADVANCED_FACE('',(#3709),#1090,.T.);
#32458=ADVANCED_FACE('',(#3710),#1091,.F.);
#32459=ADVANCED_FACE('',(#3711),#1092,.T.);
#32460=ADVANCED_FACE('',(#3712),#1093,.F.);
#32461=ADVANCED_FACE('',(#3713),#1094,.T.);
#32462=ADVANCED_FACE('',(#3714),#1095,.F.);
#32463=ADVANCED_FACE('',(#3715),#1096,.T.);
#32464=ADVANCED_FACE('',(#3716),#1097,.F.);
#32465=ADVANCED_FACE('',(#3717),#1098,.T.);
#32466=ADVANCED_FACE('',(#3718),#1099,.F.);
#32467=ADVANCED_FACE('',(#3719),#1100,.T.);
#32468=ADVANCED_FACE('',(#3720),#1101,.F.);
#32469=ADVANCED_FACE('',(#3721),#2618,.T.);
#32470=ADVANCED_FACE('',(#3722),#2129,.F.);
#32471=ADVANCED_FACE('',(#3723),#1102,.T.);
#32472=ADVANCED_FACE('',(#3724),#1103,.F.);
#32473=ADVANCED_FACE('',(#3725),#1104,.T.);
#32474=ADVANCED_FACE('',(#3726),#1105,.F.);
#32475=ADVANCED_FACE('',(#3727),#2619,.T.);
#32476=ADVANCED_FACE('',(#3728),#2130,.F.);
#34170=CLOSED_SHELL('',(#32433,#32434,#32435,#32436,#32437,#32438,#32439,
#32440,#32441,#32442,#32443,#32444,#32445,#32446,#32447,#32448,#32449,#32450,
#32451,#32452,#32453,#32454,#32455,#32456,#32457,#32458,#32459,#32460,#32461,
#32462,#32463,#32464,#32465,#32466,#32467,#32468,#32469,#32470,#32471,#32472,
#32473,#32474,#32475,#32476));
#34920=AXIS2_PLACEMENT_3D('',#71740,#40155,#40156);
#34921=AXIS2_PLACEMENT_3D('',#71741,#40157,#40158);
#34922=AXIS2_PLACEMENT_3D('',#72777,#40163,#40164);
#34923=AXIS2_PLACEMENT_3D('',#72779,#40165,#40166);
#34924=AXIS2_PLACEMENT_3D('',#72780,#40167,#40168);
#34925=AXIS2_PLACEMENT_3D('',#72860,#40171,#40172);
#34926=AXIS2_PLACEMENT_3D('',#72862,#40173,#40174);
#34927=AXIS2_PLACEMENT_3D('',#72916,#40177,#40178);
#34928=AXIS2_PLACEMENT_3D('',#72918,#40179,#40180);
#34929=AXIS2_PLACEMENT_3D('',#72919,#40181,#40182);
#34930=AXIS2_PLACEMENT_3D('',#72920,#40183,#40184);
#34931=AXIS2_PLACEMENT_3D('',#72922,#40186,#40187);
#34932=AXIS2_PLACEMENT_3D('',#72924,#40188,#40189);
#34933=AXIS2_PLACEMENT_3D('',#72925,#40190,#40191);
#34934=AXIS2_PLACEMENT_3D('',#72926,#40192,#40193);
#34935=AXIS2_PLACEMENT_3D('',#72983,#40195,#40196);
#34936=AXIS2_PLACEMENT_3D('',#72985,#40197,#40198);
#34937=AXIS2_PLACEMENT_3D('',#73006,#40201,#40202);
#34938=AXIS2_PLACEMENT_3D('',#73008,#40203,#40204);
#34939=AXIS2_PLACEMENT_3D('',#73010,#40206,#40207);
#34940=AXIS2_PLACEMENT_3D('',#73067,#40209,#40210);
#34941=AXIS2_PLACEMENT_3D('',#73142,#40212,#40213);
#34942=AXIS2_PLACEMENT_3D('',#73214,#40215,#40216);
#34943=AXIS2_PLACEMENT_3D('',#73216,#40217,#40218);
#34944=AXIS2_PLACEMENT_3D('',#73218,#40220,#40221);
#34945=AXIS2_PLACEMENT_3D('',#73275,#40223,#40224);
#34946=AXIS2_PLACEMENT_3D('',#73350,#40226,#40227);
#34947=AXIS2_PLACEMENT_3D('',#73425,#40229,#40230);
#34948=AXIS2_PLACEMENT_3D('',#73618,#40232,#40233);
#34949=AXIS2_PLACEMENT_3D('',#73626,#40234,#40235);
#34950=AXIS2_PLACEMENT_3D('',#73732,#40238,#40239);
#34951=AXIS2_PLACEMENT_3D('',#73834,#40241,#40242);
#34952=AXIS2_PLACEMENT_3D('',#73909,#40244,#40245);
#34953=AXIS2_PLACEMENT_3D('',#74020,#40247,#40248);
#34954=AXIS2_PLACEMENT_3D('',#74122,#40250,#40251);
#34955=AXIS2_PLACEMENT_3D('',#74142,#40253,#40254);
#34956=AXIS2_PLACEMENT_3D('',#74144,#40255,#40256);
#34957=AXIS2_PLACEMENT_3D('',#74146,#40258,#40259);
#34958=AXIS2_PLACEMENT_3D('',#74203,#40261,#40262);
#34959=AXIS2_PLACEMENT_3D('',#74278,#40264,#40265);
#34960=AXIS2_PLACEMENT_3D('',#74298,#40267,#40268);
#34961=AXIS2_PLACEMENT_3D('',#74300,#40270,#40271);
#40155=DIRECTION('axis',(0.,0.,1.));
#40156=DIRECTION('refdir',(1.,0.,0.));
#40157=DIRECTION('center_axis',(0.,-1.,0.));
#40158=DIRECTION('ref_axis',(0.,0.,-1.));
#40159=DIRECTION('',(0.,0.,1.));
#40160=DIRECTION('',(0.,0.,-1.));
#40161=DIRECTION('',(0.,0.,1.));
#40162=DIRECTION('',(0.,0.,-1.));
#40163=DIRECTION('center_axis',(0.,-1.,0.));
#40164=DIRECTION('ref_axis',(1.,0.,0.));
#40165=DIRECTION('center_axis',(0.,-1.,0.));
#40166=DIRECTION('ref_axis',(1.,0.,0.));
#40167=DIRECTION('center_axis',(0.,-1.,0.));
#40168=DIRECTION('ref_axis',(0.,0.,-1.));
#40169=DIRECTION('',(0.,0.,-1.));
#40170=DIRECTION('',(0.,0.,1.));
#40171=DIRECTION('center_axis',(0.,-1.,0.));
#40172=DIRECTION('ref_axis',(1.,0.,0.));
#40173=DIRECTION('center_axis',(0.,-1.,0.));
#40174=DIRECTION('ref_axis',(1.,0.,0.));
#40175=DIRECTION('',(0.,0.,1.));
#40176=DIRECTION('',(0.,0.,-1.));
#40177=DIRECTION('center_axis',(0.,-1.,0.));
#40178=DIRECTION('ref_axis',(-1.,0.,1.45603019622971E-16));
#40179=DIRECTION('center_axis',(0.,-1.,0.));
#40180=DIRECTION('ref_axis',(1.,0.,0.));
#40181=DIRECTION('center_axis',(0.,0.,1.));
#40182=DIRECTION('ref_axis',(1.,0.,0.));
#40183=DIRECTION('center_axis',(0.,-1.,0.));
#40184=DIRECTION('ref_axis',(-1.,0.,5.51957469628984E-16));
#40185=DIRECTION('',(0.,-1.,0.));
#40186=DIRECTION('center_axis',(0.,-1.,0.));
#40187=DIRECTION('ref_axis',(1.,0.,3.64007549057428E-16));
#40188=DIRECTION('center_axis',(0.,-1.,0.));
#40189=DIRECTION('ref_axis',(1.,0.,0.));
#40190=DIRECTION('center_axis',(4.55009436321785E-16,0.,-1.));
#40191=DIRECTION('ref_axis',(-1.,0.,-4.55009436321785E-16));
#40192=DIRECTION('center_axis',(0.,-1.,0.));
#40193=DIRECTION('ref_axis',(1.,0.,4.73106402539129E-16));
#40194=DIRECTION('',(0.,-1.,0.));
#40195=DIRECTION('center_axis',(0.954875323536579,7.50697958768155E-7,0.297006930054419));
#40196=DIRECTION('ref_axis',(0.210016056245524,-0.707106999787048,-0.675198450065784));
#40197=DIRECTION('center_axis',(3.24818764753068E-6,-1.23643017124277E-11,
0.999999999994725));
#40198=DIRECTION('ref_axis',(0.707106611008976,-0.707106951360347,-2.29682370226244E-6));
#40199=DIRECTION('',(0.,-1.,0.));
#40200=DIRECTION('',(0.,-1.,0.));
#40201=DIRECTION('center_axis',(0.,0.,1.));
#40202=DIRECTION('ref_axis',(-1.,0.,0.));
#40203=DIRECTION('center_axis',(0.,0.,1.));
#40204=DIRECTION('ref_axis',(3.70074341541716E-15,-1.,0.));
#40205=DIRECTION('',(0.,0.,1.));
#40206=DIRECTION('center_axis',(1.,0.,3.15544362088E-30));
#40207=DIRECTION('ref_axis',(-3.15544362088E-30,0.,1.));
#40208=DIRECTION('',(0.,-1.,0.));
#40209=DIRECTION('center_axis',(-0.999999999998532,6.19186184291188E-7,
1.59754516227631E-6));
#40210=DIRECTION('ref_axis',(6.91803843401809E-7,-0.707106972624542,0.707106589748163));
#40211=DIRECTION('',(0.,-1.,0.));
#40212=DIRECTION('center_axis',(-1.86759121106465E-6,5.22456588938859E-9,
-0.999999999998256));
#40213=DIRECTION('ref_axis',(0.70710691586452,0.707106646507323,-1.3168923360884E-6));
#40214=DIRECTION('',(0.,-1.,0.));
#40215=DIRECTION('center_axis',(0.,0.,-1.));
#40216=DIRECTION('ref_axis',(1.,0.,0.));
#40217=DIRECTION('center_axis',(-8.90823913776128E-12,8.90823913776095E-12,
-1.));
#40218=DIRECTION('ref_axis',(0.707106781186548,0.707106781186547,-2.33979865511361E-25));
#40219=DIRECTION('',(0.,0.,-1.));
#40220=DIRECTION('center_axis',(-1.,0.,0.));
#40221=DIRECTION('ref_axis',(0.,0.,1.));
#40222=DIRECTION('',(0.,-1.,0.));
#40223=DIRECTION('center_axis',(0.954873176751286,2.05613266315519E-6,-0.297013831860875));
#40224=DIRECTION('ref_axis',(0.21001907334242,0.707106892215597,0.675197624265364));
#40225=DIRECTION('',(0.,-1.,0.));
#40226=DIRECTION('center_axis',(0.223512880731291,7.41972707830334E-7,-0.974700975759566));
#40227=DIRECTION('ref_axis',(0.689217337981213,0.707107001090406,0.158047935877135));
#40228=DIRECTION('',(0.,-1.,0.));
#40229=DIRECTION('center_axis',(0.223525571185457,4.30435661235287E-6,0.974698065560658));
#40230=DIRECTION('ref_axis',(0.689215820938936,-0.707107264577136,-0.158053372471798));
#40231=DIRECTION('',(0.,-1.,0.));
#40232=DIRECTION('center_axis',(-0.999936197465094,6.12637967379869E-7,
-0.0112960612017118));
#40233=DIRECTION('ref_axis',(-0.00798708627314562,0.707106960926242,0.707061491146646));
#40234=DIRECTION('center_axis',(7.57660191412773E-6,-3.13873518338466E-6,
0.999999999966372));
#40235=DIRECTION('ref_axis',(-0.707106276301774,-0.707107286063998,3.13804024942857E-6));
#40236=DIRECTION('',(0.,-1.,0.));
#40237=DIRECTION('',(0.,-1.,0.));
#40238=DIRECTION('center_axis',(0.223393486583629,1.49897152312551E-6,-0.974728346848374));
#40239=DIRECTION('ref_axis',(0.689238163153829,-0.707105855285527,0.157962222930858));
#40240=DIRECTION('',(0.,-1.,0.));
#40241=DIRECTION('center_axis',(0.999999999997494,8.08987842812791E-7,2.08724718407666E-6));
#40242=DIRECTION('ref_axis',(-9.03865987698544E-7,-0.707106733063809,0.707106829308705));
#40243=DIRECTION('',(0.,-1.,0.));
#40244=DIRECTION('center_axis',(0.223400190145581,-3.77165381060116E-6,
0.974726810459573));
#40245=DIRECTION('ref_axis',(-0.689235920657423,-0.707107409693601,0.157965049399924));
#40246=DIRECTION('',(0.,-1.,0.));
#40247=DIRECTION('center_axis',(-0.999936145359499,-1.756468756071E-6,0.011300672568584));
#40248=DIRECTION('ref_axis',(-0.00798954026920954,-0.707106781570959,-0.707061642788411));
#40249=DIRECTION('',(0.,-1.,0.));
#40250=DIRECTION('center_axis',(0.,0.,-1.));
#40251=DIRECTION('ref_axis',(0.707106781635978,-0.707106780737117,0.));
#40252=DIRECTION('',(0.,-1.,0.));
#40253=DIRECTION('center_axis',(0.,0.,1.));
#40254=DIRECTION('ref_axis',(-1.,0.,0.));
#40255=DIRECTION('center_axis',(-3.91056427499541E-6,-3.975788198415E-10,
-0.999999999992354));
#40256=DIRECTION('ref_axis',(-0.707106338048842,0.70710722431857,2.76490365336202E-6));
#40257=DIRECTION('',(0.,0.,-1.));
#40258=DIRECTION('center_axis',(1.,0.,0.));
#40259=DIRECTION('ref_axis',(0.,1.,0.));
#40260=DIRECTION('',(0.,-1.,0.));
#40261=DIRECTION('center_axis',(-0.999999999976519,-2.47658205161019E-6,
6.38976095921973E-6));
#40262=DIRECTION('ref_axis',(-2.76704852940032E-6,-0.707105293783789,-0.707108268580764));
#40263=DIRECTION('',(0.,-1.,0.));
#40264=DIRECTION('center_axis',(0.,0.,1.));
#40265=DIRECTION('ref_axis',(0.707106781635978,0.707106780737117,0.));
#40266=DIRECTION('',(0.,-1.,0.));
#40267=DIRECTION('center_axis',(0.,0.,-1.));
#40268=DIRECTION('ref_axis',(1.,0.,0.));
#40269=DIRECTION('',(0.,0.,1.));
#40270=DIRECTION('center_axis',(-1.,0.,0.));
#40271=DIRECTION('ref_axis',(0.,0.,1.));
#71740=CARTESIAN_POINT('',(0.,0.,0.));
#71741=CARTESIAN_POINT('Origin',(-3.35265884719E-30,-42.6742356128,3.15283103411E-22));
#71742=CARTESIAN_POINT('',(0.77958411848117,-42.6742356128,-4.94563407380883));
#71743=CARTESIAN_POINT('',(6.75287820063378,-42.6742356128,2.63899277819224));
#71744=CARTESIAN_POINT('Ctrl Pts',(0.779584195372,-42.6742356128,-4.94563441411));
#71745=CARTESIAN_POINT('Ctrl Pts',(0.783019505297316,-42.6742356128,-4.96062388339205));
#71746=CARTESIAN_POINT('Ctrl Pts',(0.786509971280464,-42.6742356128,-4.97559800551016));
#71747=CARTESIAN_POINT('Ctrl Pts',(0.790056389615954,-42.6742356128,-4.99056023421706));
#71748=CARTESIAN_POINT('Ctrl Pts',(0.829308383727368,-42.6742356128,-5.15616317711285));
#71749=CARTESIAN_POINT('Ctrl Pts',(0.875381467538884,-42.6742356128,-5.32014544362963));
#71750=CARTESIAN_POINT('Ctrl Pts',(0.928124152698679,-42.6742356127999,
-5.48195135268744));
#71751=CARTESIAN_POINT('Ctrl Pts',(0.981494143503791,-42.6742356127999,
-5.64568173259634));
#71752=CARTESIAN_POINT('Ctrl Pts',(1.04169323701819,-42.6742356127997,-5.80718344510452));
#71753=CARTESIAN_POINT('Ctrl Pts',(1.1085137075534,-42.6742356127992,-5.96589766472136));
#71754=CARTESIAN_POINT('Ctrl Pts',(1.17574469865151,-42.6742356127987,-6.12558696652868));
#71755=CARTESIAN_POINT('Ctrl Pts',(1.24967852311599,-42.6742356127978,-6.28245419176864));
#71756=CARTESIAN_POINT('Ctrl Pts',(1.33005445375074,-42.6742356127966,-6.43595063967566));
#71757=CARTESIAN_POINT('Ctrl Pts',(1.41084070525712,-42.6742356127954,-6.59023069028317));
#71758=CARTESIAN_POINT('Ctrl Pts',(1.49813483665254,-42.6742356127938,-6.74110522701633));
#71759=CARTESIAN_POINT('Ctrl Pts',(1.59162503957232,-42.674235612792,-6.88804121025148));
#71760=CARTESIAN_POINT('Ctrl Pts',(1.68547908635635,-42.6742356127902,-7.03554903689125));
#71761=CARTESIAN_POINT('Ctrl Pts',(1.78557734186053,-42.6742356127882,-7.17908735951526));
#71762=CARTESIAN_POINT('Ctrl Pts',(1.89155970140233,-42.6742356127863,-7.31814464429339));
#71763=CARTESIAN_POINT('Ctrl Pts',(1.99789293179152,-42.6742356127845,-7.45766229952898));
#71764=CARTESIAN_POINT('Ctrl Pts',(2.11014909709696,-42.6742356127828,-7.5926689596614));
#71765=CARTESIAN_POINT('Ctrl Pts',(2.22792250961881,-42.6742356127818,-7.72267943330251));
#71766=CARTESIAN_POINT('Ctrl Pts',(2.34573059330044,-42.6742356127807,-7.8527281805557));
#71767=CARTESIAN_POINT('Ctrl Pts',(2.46905895621691,-42.6742356127804,-7.97777757592768));
#71768=CARTESIAN_POINT('Ctrl Pts',(2.59746272145967,-42.674235612781,-8.09737684660448));
#71769=CARTESIAN_POINT('Ctrl Pts',(2.72562676191173,-42.6742356127816,-8.21675283013642));
#71770=CARTESIAN_POINT('Ctrl Pts',(2.85884704246923,-42.6742356127832,-8.33069881216825));
#71771=CARTESIAN_POINT('Ctrl Pts',(2.99664585191555,-42.6742356127857,-8.4388044646528));
#71772=CARTESIAN_POINT('Ctrl Pts',(3.11571505661626,-42.6742356127878,-8.53221640425306));
#71773=CARTESIAN_POINT('Ctrl Pts',(3.23820210993358,-42.6742356127905,-8.62126826774772));
#71774=CARTESIAN_POINT('Ctrl Pts',(3.363779477155,-42.6742356127932,-8.70572001193011));
#71775=CARTESIAN_POINT('Ctrl Pts',(3.50872753999223,-42.6742356127963,-8.80319869772609));
#71776=CARTESIAN_POINT('Ctrl Pts',(3.65779162004941,-42.6742356127977,-8.89454681427974));
#71777=CARTESIAN_POINT('Ctrl Pts',(3.81044289926437,-42.6742356127985,-8.97943725563266));
#71778=CARTESIAN_POINT('Ctrl Pts',(3.96182994811744,-42.6742356127994,-9.06362464966135));
#71779=CARTESIAN_POINT('Ctrl Pts',(4.11674479055607,-42.6742356127997,-9.14146074594292));
#71780=CARTESIAN_POINT('Ctrl Pts',(4.27464700945189,-42.6742356127998,-9.21267133077376));
#71781=CARTESIAN_POINT('Ctrl Pts',(4.43163594214289,-42.6742356128,-9.28347004270492));
#71782=CARTESIAN_POINT('Ctrl Pts',(4.59157758029576,-42.6742356128,-9.34771951000529));
#71783=CARTESIAN_POINT('Ctrl Pts',(4.75391970062592,-42.6742356128,-9.4051969786154));
#71784=CARTESIAN_POINT('Ctrl Pts',(4.91468786119625,-42.6742356128,-9.46211718443686));
#71785=CARTESIAN_POINT('Ctrl Pts',(5.07780996923672,-42.6742356128,-9.51239595479921));
#71786=CARTESIAN_POINT('Ctrl Pts',(5.24273211710097,-42.6742356128,-9.55586484972988));
#71787=CARTESIAN_POINT('Ctrl Pts',(5.32221123857816,-42.6742356128,-9.57681333739765));
#71788=CARTESIAN_POINT('Ctrl Pts',(5.40210816909334,-42.6742356128,-9.59618098515424));
#71789=CARTESIAN_POINT('Ctrl Pts',(5.48235965328664,-42.6742356128,-9.61395309319581));
#71790=CARTESIAN_POINT('Ctrl Pts',(5.64903325566381,-42.6742356128,-9.65086382822956));
#71791=CARTESIAN_POINT('Ctrl Pts',(5.8172324747726,-42.6742356128,-9.68088796096779));
#71792=CARTESIAN_POINT('Ctrl Pts',(5.9863825361148,-42.6742356128,-9.70391857948388));
#71793=CARTESIAN_POINT('Ctrl Pts',(6.15680323563844,-42.6742356128,-9.72712220168082));
#71794=CARTESIAN_POINT('Ctrl Pts',(6.32818887600278,-42.6742356128,-9.74322687290936));
#71795=CARTESIAN_POINT('Ctrl Pts',(6.4999462288075,-42.6742356128,-9.75217621766798));
#71796=CARTESIAN_POINT('Ctrl Pts',(6.67284585238956,-42.6742356128,-9.7611850799659));
#71797=CARTESIAN_POINT('Ctrl Pts',(6.84612189524726,-42.6742356128,-9.76294316381342));
#71798=CARTESIAN_POINT('Ctrl Pts',(7.01916749716638,-42.6742356128,-9.75744593352396));
#71799=CARTESIAN_POINT('Ctrl Pts',(7.19318017371352,-42.6742356128,-9.75191798166816));
#71800=CARTESIAN_POINT('Ctrl Pts',(7.3669595611434,-42.6742356128,-9.73905344497));
#71801=CARTESIAN_POINT('Ctrl Pts',(7.53989075903008,-42.6742356128,-9.71890043121172));
#71802=CARTESIAN_POINT('Ctrl Pts',(7.71357133496519,-42.6742356128,-9.69866008661722));
#71803=CARTESIAN_POINT('Ctrl Pts',(7.88639608023403,-42.6742356128,-9.67106802306371));
#71804=CARTESIAN_POINT('Ctrl Pts',(8.05774833885344,-42.6742356128,-9.63622514593106));
#71805=CARTESIAN_POINT('Ctrl Pts',(8.23576088873995,-42.6742356128,-9.60002796094069));
#71806=CARTESIAN_POINT('Ctrl Pts',(8.41218387461858,-42.6742356128,-9.5560050970399));
#71807=CARTESIAN_POINT('Ctrl Pts',(8.5863377901713,-42.6742356128,-9.50432770550163));
#71808=CARTESIAN_POINT('Ctrl Pts',(8.75375175092122,-42.6742356128,-9.45465028784963));
#71809=CARTESIAN_POINT('Ctrl Pts',(8.91907037676882,-42.6742356128,-9.39789907292805));
#71810=CARTESIAN_POINT('Ctrl Pts',(9.08169780495813,-42.6742356128,-9.33427897488519));
#71811=CARTESIAN_POINT('Ctrl Pts',(9.24517506010802,-42.6742356128,-9.27032642323869));
#71812=CARTESIAN_POINT('Ctrl Pts',(9.4059329078901,-42.6742356128,-9.19943320191932));
#71813=CARTESIAN_POINT('Ctrl Pts',(9.56339297670855,-42.6742356128,-9.12185394747491));
#71814=CARTESIAN_POINT('Ctrl Pts',(9.72049523523666,-42.6742356128,-9.04445098315768));
#71815=CARTESIAN_POINT('Ctrl Pts',(9.87431442098647,-42.6742356128,-8.96039245709044));
#71816=CARTESIAN_POINT('Ctrl Pts',(10.0242991772771,-42.6742356128,-8.86997765445494));
#71817=CARTESIAN_POINT('Ctrl Pts',(10.1737494126108,-42.6742356128,-8.77988507527749));
#71818=CARTESIAN_POINT('Ctrl Pts',(10.3193922472071,-42.6742356128,-8.68348157024173));
#71819=CARTESIAN_POINT('Ctrl Pts',(10.4607090001088,-42.6742356128,-8.58110749092089));
#71820=CARTESIAN_POINT('Ctrl Pts',(10.6009930196497,-42.6742356128,-8.47948155451174));
#71821=CARTESIAN_POINT('Ctrl Pts',(10.737013731518,-42.6742356128,-8.37197213719144));
#71822=CARTESIAN_POINT('Ctrl Pts',(10.8682937302911,-42.6742356128,-8.25895379645599));
#71823=CARTESIAN_POINT('Ctrl Pts',(10.9988863407824,-42.6742356128,-8.14652722509724));
#71824=CARTESIAN_POINT('Ctrl Pts',(11.124787528533,-42.6742356128,-8.02864939656428));
#71825=CARTESIAN_POINT('Ctrl Pts',(11.2455604901236,-42.6742356128,-7.90572832483952));
#71826=CARTESIAN_POINT('Ctrl Pts',(11.3653029051114,-42.6742356128,-7.78385612937986));
#71827=CARTESIAN_POINT('Ctrl Pts',(11.4800040444459,-42.6742356128,-7.65702653237569));
#71828=CARTESIAN_POINT('Ctrl Pts',(11.5892739367748,-42.6742356128,-7.52567390389989));
#71829=CARTESIAN_POINT('Ctrl Pts',(11.6246642014889,-42.6742356128,-7.48313149634753));
#71830=CARTESIAN_POINT('Ctrl Pts',(11.659485033899,-42.6742356128,-7.44011491296741));
#71831=CARTESIAN_POINT('Ctrl Pts',(11.6937240507251,-42.6742356128,-7.39663970957412));
#71832=CARTESIAN_POINT('Ctrl Pts',(11.7994911640488,-42.6742356128,-7.26234126323053));
#71833=CARTESIAN_POINT('Ctrl Pts',(11.8997014351145,-42.6742356128,-7.12366634871067));
#71834=CARTESIAN_POINT('Ctrl Pts',(11.994008150501,-42.6742356128,-6.98108829107189));
#71835=CARTESIAN_POINT('Ctrl Pts',(12.0890003774915,-42.6742356128,-6.83747383944364));
#71836=CARTESIAN_POINT('Ctrl Pts',(12.1780028286506,-42.6742356128,-6.68989952409289));
#71837=CARTESIAN_POINT('Ctrl Pts',(12.2607064520845,-42.6742356128,-6.53887699905973));
#71838=CARTESIAN_POINT('Ctrl Pts',(12.3439374138085,-42.6742356128,-6.38689151790917));
#71839=CARTESIAN_POINT('Ctrl Pts',(12.420788886891,-42.6742356128,-6.23141395914406));
#71840=CARTESIAN_POINT('Ctrl Pts',(12.4909927754262,-42.6742356128,-6.07299041838974));
#71841=CARTESIAN_POINT('Ctrl Pts',(12.5615678727858,-42.6742356128,-5.91372920015702));
#71842=CARTESIAN_POINT('Ctrl Pts',(12.6254248272806,-42.6742356128,-5.75149102399791));
#71843=CARTESIAN_POINT('Ctrl Pts',(12.6823396578243,-42.6742356128,-5.58685163845662));
#71844=CARTESIAN_POINT('Ctrl Pts',(12.7394829364501,-42.6742356128,-5.42155141370174));
#71845=CARTESIAN_POINT('Ctrl Pts',(12.7896281850343,-42.6742356128,-5.25383093843157));
#71846=CARTESIAN_POINT('Ctrl Pts',(12.8325983909053,-42.6742356128,-5.08428994230337));
#71847=CARTESIAN_POINT('Ctrl Pts',(12.87720466428,-42.6742356128,-4.90829376382998));
#71848=CARTESIAN_POINT('Ctrl Pts',(12.9140787347158,-42.6742356128,-4.73033603312672));
#71849=CARTESIAN_POINT('Ctrl Pts',(12.9430798859501,-42.6742356128,-4.55110211074482));
#71850=CARTESIAN_POINT('Ctrl Pts',(12.9710073007924,-42.6742356128,-4.37850413131527));
#71851=CARTESIAN_POINT('Ctrl Pts',(12.9916343265915,-42.6742356128,-4.20472180630914));
#71852=CARTESIAN_POINT('Ctrl Pts',(13.0048866885129,-42.6742356128,-4.03038094709754));
#71853=CARTESIAN_POINT('Ctrl Pts',(13.0181761619694,-42.6742356128,-3.85555186873162));
#71854=CARTESIAN_POINT('Ctrl Pts',(13.0240497216501,-42.6742356128,-3.68016120196708));
#71855=CARTESIAN_POINT('Ctrl Pts',(13.0224853990129,-42.6742356128,-3.50483862976804));
#71856=CARTESIAN_POINT('Ctrl Pts',(13.0209250079126,-42.6742356128,-3.32995668735456));
#71857=CARTESIAN_POINT('Ctrl Pts',(13.0119640639272,-42.6742356128,-3.15514278510275));
#71858=CARTESIAN_POINT('Ctrl Pts',(12.9956325370699,-42.6742356128,-2.9810213883885));
#71859=CARTESIAN_POINT('Ctrl Pts',(12.9793624016983,-42.6742356128,-2.80755452761145));
#71860=CARTESIAN_POINT('Ctrl Pts',(12.9557769932041,-42.6742356128,-2.63477525560034));
#71861=CARTESIAN_POINT('Ctrl Pts',(12.9249574485041,-42.6742356128,-2.46329630674595));
#71862=CARTESIAN_POINT('Ctrl Pts',(12.8943693323404,-42.6742356128,-2.29310501877498));
#71863=CARTESIAN_POINT('Ctrl Pts',(12.8566553491569,-42.6742356128,-2.12419486156537));
#71864=CARTESIAN_POINT('Ctrl Pts',(12.8119453525895,-42.6742356128,-1.95715618241776));
#71865=CARTESIAN_POINT('Ctrl Pts',(12.7674725431208,-42.6742356128,-1.79100364558063));
#71866=CARTESIAN_POINT('Ctrl Pts',(12.7160777651395,-42.6742356128,-1.62670303780744));
#71867=CARTESIAN_POINT('Ctrl Pts',(12.6579386831089,-42.6742356128,-1.46482287587078));
#71868=CARTESIAN_POINT('Ctrl Pts',(12.6002987770892,-42.6742356128,-1.30433259988757));
#71869=CARTESIAN_POINT('Ctrl Pts',(12.5360299222692,-42.6742356128,-1.14622161782475));
#71870=CARTESIAN_POINT('Ctrl Pts',(12.4653539433873,-42.6742356128,-0.991028010976763));
#71871=CARTESIAN_POINT('Ctrl Pts',(12.4420672694898,-42.6742356128,-0.939894047630111));
#71872=CARTESIAN_POINT('Ctrl Pts',(12.4180854288606,-42.6742356128,-0.889076651319818));
#71873=CARTESIAN_POINT('Ctrl Pts',(12.3934175172357,-42.6742356128,-0.838594619595771));
#71874=CARTESIAN_POINT('Ctrl Pts',(12.3185024105953,-42.6742356128,-0.685283433487476));
#71875=CARTESIAN_POINT('Ctrl Pts',(12.2372578125187,-42.6742356128,-0.535070520939901));
#71876=CARTESIAN_POINT('Ctrl Pts',(12.1499565739039,-42.6742356128,-0.388469222689598));
#71877=CARTESIAN_POINT('Ctrl Pts',(12.061958185551,-42.6742356128,-0.240697230205108));
#71878=CARTESIAN_POINT('Ctrl Pts',(11.9678062121948,-42.6742356128,-0.0965949378574854));
#71879=CARTESIAN_POINT('Ctrl Pts',(11.8678252730607,-42.6742356128,0.0433402117257184));
#71880=CARTESIAN_POINT('Ctrl Pts',(11.7671342669587,-42.6742356128,0.184269184013886));
#71881=CARTESIAN_POINT('Ctrl Pts',(11.660531396595,-42.6742356128,0.320971434223083));
#71882=CARTESIAN_POINT('Ctrl Pts',(11.5483911271814,-42.6742356128,0.452970093455365));
#71883=CARTESIAN_POINT('Ctrl Pts',(11.4355782693087,-42.6742356128,0.585760446655333));
#71884=CARTESIAN_POINT('Ctrl Pts',(11.3171615973516,-42.6742356128,0.713790436676404));
#71885=CARTESIAN_POINT('Ctrl Pts',(11.1935625752031,-42.6742356128,0.836608787067195));
#71886=CARTESIAN_POINT('Ctrl Pts',(11.0693854080758,-42.6742356128,0.960001630777979));
#71887=CARTESIAN_POINT('Ctrl Pts',(10.9399775204536,-42.6742356128,1.0781337847633));
#71888=CARTESIAN_POINT('Ctrl Pts',(10.805803514957,-42.6742356128,1.1905847691352));
#71889=CARTESIAN_POINT('Ctrl Pts',(10.6669174748723,-42.6742356128,1.30698490092859));
#71890=CARTESIAN_POINT('Ctrl Pts',(10.5229247523534,-42.6742356128,1.41729739891248));
#71891=CARTESIAN_POINT('Ctrl Pts',(10.3743783545598,-42.6742356128,1.52110055406783));
#71892=CARTESIAN_POINT('Ctrl Pts',(10.2308082149157,-42.6742356128,1.62142633579327));
#71893=CARTESIAN_POINT('Ctrl Pts',(10.0829839466795,-42.6742356128,1.71567215095053));
#71894=CARTESIAN_POINT('Ctrl Pts',(9.93143848173256,-42.6742356128,1.80349800771626));
#71895=CARTESIAN_POINT('Ctrl Pts',(9.77978308346317,-42.6742356128,1.89138757465791));
#71896=CARTESIAN_POINT('Ctrl Pts',(9.62440150387112,-42.6742356128,1.97284768977086));
#71897=CARTESIAN_POINT('Ctrl Pts',(9.46585194695658,-42.6742356128,2.04758417096211));
#71898=CARTESIAN_POINT('Ctrl Pts',(9.30767676126653,-42.6742356128,2.12214418248343));
#71899=CARTESIAN_POINT('Ctrl Pts',(9.14634881129091,-42.6742356128,2.19001213657793));
#71900=CARTESIAN_POINT('Ctrl Pts',(8.98244418750696,-42.6742356128,2.25094289839676));
#71901=CARTESIAN_POINT('Ctrl Pts',(8.81914713258895,-42.6742356128,2.31164779938869));
#71902=CARTESIAN_POINT('Ctrl Pts',(8.65329273944362,-42.6742356128,2.36546671959078));
#71903=CARTESIAN_POINT('Ctrl Pts',(8.48546838207095,-42.6742356128,2.41220585261861));
#71904=CARTESIAN_POINT('Ctrl Pts',(8.31891495058699,-42.6742356128,2.45859103241158));
#71905=CARTESIAN_POINT('Ctrl Pts',(8.15042154522815,-42.6742356128,2.49800316356433));
#71906=CARTESIAN_POINT('Ctrl Pts',(7.98057573186983,-42.6742356128,2.53030228157987));
#71907=CARTESIAN_POINT('Ctrl Pts',(7.8116501798998,-42.6742356128,2.56242639598126));
#71908=CARTESIAN_POINT('Ctrl Pts',(7.64138708606372,-42.6742356128,2.58751427080524));
#71909=CARTESIAN_POINT('Ctrl Pts',(7.47037401862466,-42.6742356128,2.60547871329712));
#71910=CARTESIAN_POINT('Ctrl Pts',(7.30086061566379,-42.6742356128,2.62328562024696));
#71911=CARTESIAN_POINT('Ctrl Pts',(7.13061057599309,-42.6742356128,2.63409341996058));
#71912=CARTESIAN_POINT('Ctrl Pts',(6.96020184664722,-42.6742356128,2.63786809596414));
#71913=CARTESIAN_POINT('Ctrl Pts',(6.90647999391455,-42.6742356128,2.63905807366748));
#71914=CARTESIAN_POINT('Ctrl Pts',(6.85274239824904,-42.6742356128,2.63954945473006));
#71915=CARTESIAN_POINT('Ctrl Pts',(6.79900722782363,-42.6742356128,2.63934225086415));
#71916=CARTESIAN_POINT('Ctrl Pts',(6.78363056283946,-42.6742356128,2.63928295814387));
#71917=CARTESIAN_POINT('Ctrl Pts',(6.76825498579667,-42.6742356128,2.63916647454667));
#71918=CARTESIAN_POINT('Ctrl Pts',(6.75287834563,-42.6742356128,2.63899277983));
#71919=CARTESIAN_POINT('',(5.94384247274,-42.6742356128,3.43894307771));
#71920=CARTESIAN_POINT('Ctrl Pts',(6.75287805523922,-42.6742356128,2.63899277654992));
#71921=CARTESIAN_POINT('Ctrl Pts',(6.71005222967492,-42.6742356128,2.63850906375133));
#71922=CARTESIAN_POINT('Ctrl Pts',(6.66724147238406,-42.6742356127937,2.64150712921468));
#71923=CARTESIAN_POINT('Ctrl Pts',(6.62496447000998,-42.6742356127904,2.64789261444747));
#71924=CARTESIAN_POINT('Ctrl Pts',(6.60814536827622,-42.674235612789,2.65043295836305));
#71925=CARTESIAN_POINT('Ctrl Pts',(6.59141084641839,-42.6742356127902,2.65350887060177));
#71926=CARTESIAN_POINT('Ctrl Pts',(6.57479370413688,-42.6742356127937,2.65711208455179));
#71927=CARTESIAN_POINT('Ctrl Pts',(6.53437461602468,-42.6742356128024,2.66587644485308));
#71928=CARTESIAN_POINT('Ctrl Pts',(6.49464930529023,-42.6742356128,2.67776791556408));
#71929=CARTESIAN_POINT('Ctrl Pts',(6.45607632377881,-42.6742356128,2.69263942998386));
#71930=CARTESIAN_POINT('Ctrl Pts',(6.4387274004743,-42.6742356128,2.69932817306207));
#71931=CARTESIAN_POINT('Ctrl Pts',(6.42161145731401,-42.6742356128,2.70661910716981));
#71932=CARTESIAN_POINT('Ctrl Pts',(6.40476925681742,-42.6742356128,2.71449546272456));
#71933=CARTESIAN_POINT('Ctrl Pts',(6.37094623967965,-42.6742356128,2.73031299850116));
#71934=CARTESIAN_POINT('Ctrl Pts',(6.33822887458183,-42.6742356128,2.74849417854391));
#71935=CARTESIAN_POINT('Ctrl Pts',(6.30693936358219,-42.6742356128,2.76887107730016));
#71936=CARTESIAN_POINT('Ctrl Pts',(6.27647408768983,-42.6742356128,2.7887112033554));
#71937=CARTESIAN_POINT('Ctrl Pts',(6.2473622386234,-42.6742356128,2.81063362727969));
#71938=CARTESIAN_POINT('Ctrl Pts',(6.21988117165712,-42.6742356128,2.8344393996307));
#71939=CARTESIAN_POINT('Ctrl Pts',(6.19315655162769,-42.6742356128,2.85758989161735));
#71940=CARTESIAN_POINT('Ctrl Pts',(6.16797397175328,-42.6742356128,2.88252167936477));
#71941=CARTESIAN_POINT('Ctrl Pts',(6.14455644811797,-42.6742356128,2.90901447161481));
#71942=CARTESIAN_POINT('Ctrl Pts',(6.13747930837076,-42.6742356128,2.91702100535285));
#71943=CARTESIAN_POINT('Ctrl Pts',(6.13056316699852,-42.6742356128,2.92516982658604));
#71944=CARTESIAN_POINT('Ctrl Pts',(6.12381360086615,-42.6742356128,2.93345409605156));
#71945=CARTESIAN_POINT('Ctrl Pts',(6.10030182744432,-42.6742356128,2.96231193118036));
#71946=CARTESIAN_POINT('Ctrl Pts',(6.07881363705799,-42.6742356128,2.99281698557839));
#71947=CARTESIAN_POINT('Ctrl Pts',(6.05955270585133,-42.6742356127995,3.02466607617447));
#71948=CARTESIAN_POINT('Ctrl Pts',(6.04782749794023,-42.6742356127992,3.04405440195226));
#71949=CARTESIAN_POINT('Ctrl Pts',(6.0369266122408,-42.6742356127987,3.06394048669793));
#71950=CARTESIAN_POINT('Ctrl Pts',(6.02688710892239,-42.6742356127981,3.08425307204228));
#71951=CARTESIAN_POINT('Ctrl Pts',(6.00904145899223,-42.674235612797,3.12035956812436));
#71952=CARTESIAN_POINT('Ctrl Pts',(5.99392153004012,-42.6742356127982,3.15781104852967));
#71953=CARTESIAN_POINT('Ctrl Pts',(5.98169008790022,-42.6742356127991,3.19619179415814));
#71954=CARTESIAN_POINT('Ctrl Pts',(5.97574243389594,-42.6742356127994,3.21485479340334));
#71955=CARTESIAN_POINT('Ctrl Pts',(5.97047696570253,-42.6742356127997,3.23373721697366));
#71956=CARTESIAN_POINT('Ctrl Pts',(5.96590837847632,-42.6742356127998,3.25278961905919));
#71957=CARTESIAN_POINT('Ctrl Pts',(5.95476050483813,-42.6742356128001,3.29927965206879));
#71958=CARTESIAN_POINT('Ctrl Pts',(5.94776475136862,-42.6742356128,3.34678324157907));
#71959=CARTESIAN_POINT('Ctrl Pts',(5.94508590943863,-42.6742356128,3.39458200052585));
#71960=CARTESIAN_POINT('Ctrl Pts',(5.94440568849322,-42.6742356128,3.40671922916792));
#71961=CARTESIAN_POINT('Ctrl Pts',(5.9440036024013,-42.6742356128,3.4188753187901));
#71962=CARTESIAN_POINT('Ctrl Pts',(5.94388199529069,-42.6742356128,3.43103814870507));
#71963=CARTESIAN_POINT('Ctrl Pts',(5.9438556543113,-42.6742356128,3.4336727056029));
#71964=CARTESIAN_POINT('Ctrl Pts',(5.94384247124667,-42.6742356128,3.43630890719333));
#71965=CARTESIAN_POINT('Ctrl Pts',(5.94384247373,-42.6742356128,3.43894307771));
#71966=CARTESIAN_POINT('',(5.94384247076,-42.6742356128,6.92091963994));
#71967=CARTESIAN_POINT('',(5.94384247076,-42.6742356128,1.43032185727));
#71968=CARTESIAN_POINT('',(-1.17395376824544E-6,-42.6742356128,12.8643459956148));
#71969=CARTESIAN_POINT('Ctrl Pts',(5.94384247076,-42.6742356128,6.92091963994));
#71970=CARTESIAN_POINT('Ctrl Pts',(5.94384247076,-42.6742356128,7.08559459645875));
#71971=CARTESIAN_POINT('Ctrl Pts',(5.9370146386167,-42.6742356128,7.25027218802812));
#71972=CARTESIAN_POINT('Ctrl Pts',(5.92336859551397,-42.6742356128,7.41437712494407));
#71973=CARTESIAN_POINT('Ctrl Pts',(5.90973331659169,-42.6742356128,7.57835261370136));
#71974=CARTESIAN_POINT('Ctrl Pts',(5.88929072702028,-42.6742356128,7.74175617845836));
#71975=CARTESIAN_POINT('Ctrl Pts',(5.86210332732502,-42.6742356128,7.90402225667837));
#71976=CARTESIAN_POINT('Ctrl Pts',(5.8347466327406,-42.6742356128,8.06729875950804));
#71977=CARTESIAN_POINT('Ctrl Pts',(5.8005609575781,-42.6742356128,8.2294233768324));
#71978=CARTESIAN_POINT('Ctrl Pts',(5.75966185673292,-42.6742356128,8.38983112480323));
#71979=CARTESIAN_POINT('Ctrl Pts',(5.71852924283062,-42.6742356128,8.55115471940251));
#71980=CARTESIAN_POINT('Ctrl Pts',(5.67060642398137,-42.6742356128,8.71074158795276));
#71981=CARTESIAN_POINT('Ctrl Pts',(5.61606181116267,-42.6742356128,8.86803122028198));
#71982=CARTESIAN_POINT('Ctrl Pts',(5.56110091309423,-42.6742356128,9.02652128929028));
#71983=CARTESIAN_POINT('Ctrl Pts',(5.49941685038436,-42.6742356128,9.18267871222936));
#71984=CARTESIAN_POINT('Ctrl Pts',(5.43123200188617,-42.6742356128,9.33594751367258));
#71985=CARTESIAN_POINT('Ctrl Pts',(5.36281588859205,-42.6742356128,9.48973616195672));
#71986=CARTESIAN_POINT('Ctrl Pts',(5.28785494664489,-42.6742356128,9.64061635566827));
#71987=CARTESIAN_POINT('Ctrl Pts',(5.20662234382798,-42.6742356128,9.78804708151671));
#71988=CARTESIAN_POINT('Ctrl Pts',(5.12505400163844,-42.6742356128,9.93608714767537));
#71989=CARTESIAN_POINT('Ctrl Pts',(5.03716217715285,-42.6742356128,10.0806489597359));
#71990=CARTESIAN_POINT('Ctrl Pts',(4.94327034299726,-42.6742356128,10.2212087007409));
#71991=CARTESIAN_POINT('Ctrl Pts',(4.85945762028116,-42.6742356128,10.3466796184606));
#71992=CARTESIAN_POINT('Ctrl Pts',(4.77086463695177,-42.6742356128,10.4689618047329));
#71993=CARTESIAN_POINT('Ctrl Pts',(4.67775153908735,-42.6742356128,10.5877007524186));
#71994=CARTESIAN_POINT('Ctrl Pts',(4.57326078712055,-42.6742356128,10.7209486221168));
#71995=CARTESIAN_POINT('Ctrl Pts',(4.46307651478612,-42.6742356128,10.8497345855174));
#71996=CARTESIAN_POINT('Ctrl Pts',(4.3476020380169,-42.6742356128,10.9735884555489));
#71997=CARTESIAN_POINT('Ctrl Pts',(4.2318482698802,-42.6742356128,11.0977418836965));
#71998=CARTESIAN_POINT('Ctrl Pts',(4.11077889784178,-42.6742356128,11.2169391224151));
#71999=CARTESIAN_POINT('Ctrl Pts',(3.98483832342394,-42.6742356128,11.3307424063621));
#72000=CARTESIAN_POINT('Ctrl Pts',(3.85880408066675,-42.6742356128,11.4446303315351));
#72001=CARTESIAN_POINT('Ctrl Pts',(3.72789162138932,-42.6742356128,11.5531160747408));
#72002=CARTESIAN_POINT('Ctrl Pts',(3.5925810591973,-42.6742356128,11.6557998098278));
#72003=CARTESIAN_POINT('Ctrl Pts',(3.45755287962789,-42.6742356128,11.7582692519435));
#72004=CARTESIAN_POINT('Ctrl Pts',(3.3181451832739,-42.6742356128,11.8549606973954));
#72005=CARTESIAN_POINT('Ctrl Pts',(3.17486600574486,-42.6742356128,11.9455183814792));
#72006=CARTESIAN_POINT('Ctrl Pts',(3.03203906481474,-42.6742356128,12.035790235481));
#72007=CARTESIAN_POINT('Ctrl Pts',(2.88536529209994,-42.6742356128,12.1199668191166));
#72008=CARTESIAN_POINT('Ctrl Pts',(2.73537496462231,-42.6742356128,12.1977396617275));
#72009=CARTESIAN_POINT('Ctrl Pts',(2.58605108794698,-42.6742356128,12.2751669368992));
#72010=CARTESIAN_POINT('Ctrl Pts',(2.43344031083315,-42.6742356128,12.3462470988987));
#72011=CARTESIAN_POINT('Ctrl Pts',(2.27808900582438,-42.6742356128,12.4107217696588));
#72012=CARTESIAN_POINT('Ctrl Pts',(2.12360328779087,-42.6742356128,12.4748372002102));
#72013=CARTESIAN_POINT('Ctrl Pts',(1.96640773805164,-42.6742356128,12.5324204058701));
#72014=CARTESIAN_POINT('Ctrl Pts',(1.80705892470451,-42.6742356128,12.583265045202));
#72015=CARTESIAN_POINT('Ctrl Pts',(1.64933517642864,-42.6742356128,12.6335911626466));
#72016=CARTESIAN_POINT('Ctrl Pts',(1.48950209987098,-42.6742356128,12.6773153642981));
#72017=CARTESIAN_POINT('Ctrl Pts',(1.32811474567441,-42.6742356128,12.7142860970285));
#72018=CARTESIAN_POINT('Ctrl Pts',(1.16777537817361,-42.6742356128,12.7510167562027));
#72019=CARTESIAN_POINT('Ctrl Pts',(1.00590207237904,-42.6742356128,12.7810812575043));
#72020=CARTESIAN_POINT('Ctrl Pts',(0.843050953735733,-42.6742356128,12.8043806957307));
#72021=CARTESIAN_POINT('Ctrl Pts',(0.681964641973335,-42.6742356128,12.8274276394748));
#72022=CARTESIAN_POINT('Ctrl Pts',(0.519921807453605,-42.6742356128,12.8438552832061));
#72023=CARTESIAN_POINT('Ctrl Pts',(0.357469083900356,-42.6742356128,12.8536179859801));
#72024=CARTESIAN_POINT('Ctrl Pts',(0.246023068049313,-42.6742356128,12.8603154072625));
#72025=CARTESIAN_POINT('Ctrl Pts',(0.134384321199348,-42.6742356128,12.8638771742974));
#72026=CARTESIAN_POINT('Ctrl Pts',(0.0227308830019703,-42.6742356128,12.8643026885943));
#72027=CARTESIAN_POINT('Ctrl Pts',(0.015153784542996,-42.6742356128,12.8643315651231));
#72028=CARTESIAN_POINT('Ctrl Pts',(0.00757664450181249,-42.6742356128,12.8643459888667));
#72029=CARTESIAN_POINT('Ctrl Pts',(-1.17395376619811E-6,-42.6742356128,
12.8643459882));
#72030=CARTESIAN_POINT('',(-5.94384246090667,-42.6742356128,6.92091847055));
#72031=CARTESIAN_POINT('Ctrl Pts',(-1.17395377015422E-6,-42.6742356128,
12.8643460035999));
#72032=CARTESIAN_POINT('Ctrl Pts',(-0.164706854594312,-42.6742356128,12.8643460048832));
#72033=CARTESIAN_POINT('Ctrl Pts',(-0.329412989973873,-42.6742356128,12.8575186542237));
#72034=CARTESIAN_POINT('Ctrl Pts',(-0.493544656307221,-42.6742356128,12.8438731963528));
#72035=CARTESIAN_POINT('Ctrl Pts',(-0.657503591528626,-42.6742356128,12.8302420988741));
#72036=CARTESIAN_POINT('Ctrl Pts',(-0.820889093836288,-42.6742356128,12.8098073874254));
#72037=CARTESIAN_POINT('Ctrl Pts',(-0.983136337600976,-42.6742356128,12.7826312009108));
#72038=CARTESIAN_POINT('Ctrl Pts',(-1.14639445651254,-42.6742356128,12.7552856942221));
#72039=CARTESIAN_POINT('Ctrl Pts',(-1.30849990009775,-42.6742356128,12.721114535931));
#72040=CARTESIAN_POINT('Ctrl Pts',(-1.46888834825522,-42.6742356128,12.6802329315353));
#72041=CARTESIAN_POINT('Ctrl Pts',(-1.63019316272522,-42.6742356128,12.6391177534285));
#72042=CARTESIAN_POINT('Ctrl Pts',(-1.78976110989173,-42.6742356128,12.5912153307976));
#72043=CARTESIAN_POINT('Ctrl Pts',(-1.94703226892316,-42.6742356128,12.536693743442));
#72044=CARTESIAN_POINT('Ctrl Pts',(-2.10550497071265,-42.6742356128,12.4817556142433));
#72045=CARTESIAN_POINT('Ctrl Pts',(-2.26164544450545,-42.6742356128,12.4200968838488));
#72046=CARTESIAN_POINT('Ctrl Pts',(-2.41489822703504,-42.6742356128,12.3519396246491));
#72047=CARTESIAN_POINT('Ctrl Pts',(-2.56867137509239,-42.6742356128,12.2835509393861));
#72048=CARTESIAN_POINT('Ctrl Pts',(-2.71953698323308,-42.6742356128,12.2086196487733));
#72049=CARTESIAN_POINT('Ctrl Pts',(-2.86695447501242,-42.6742356128,12.1274186462476));
#72050=CARTESIAN_POINT('Ctrl Pts',(-3.01498232800051,-42.6742356128,12.045881442492));
#72051=CARTESIAN_POINT('Ctrl Pts',(-3.15953323881548,-42.6742356128,11.9580226293889));
#72052=CARTESIAN_POINT('Ctrl Pts',(-3.30008374997782,-42.6742356128,11.8641654454777));
#72053=CARTESIAN_POINT('Ctrl Pts',(-3.42578603376579,-42.6742356128,11.7802236492509));
#72054=CARTESIAN_POINT('Ctrl Pts',(-3.54828872501526,-42.6742356128,11.6914846190643));
#72055=CARTESIAN_POINT('Ctrl Pts',(-3.66723551076089,-42.6742356128,11.5982098808653));
#72056=CARTESIAN_POINT('Ctrl Pts',(-3.80048768009197,-42.6742356128,11.4937172614902));
#72057=CARTESIAN_POINT('Ctrl Pts',(-3.92927735398716,-42.6742356128,11.3835310608653));
#72058=CARTESIAN_POINT('Ctrl Pts',(-4.05313446008693,-42.6742356128,11.268054647639));
#72059=CARTESIAN_POINT('Ctrl Pts',(-4.17729331738431,-42.6742356128,11.1522969009706));
#72060=CARTESIAN_POINT('Ctrl Pts',(-4.29649533405885,-42.6742356128,11.031223354757));
#72061=CARTESIAN_POINT('Ctrl Pts',(-4.41030279594079,-42.6742356128,10.905278524681));
#72062=CARTESIAN_POINT('Ctrl Pts',(-4.52419722051319,-42.6742356128,10.7792374574946));
#72063=CARTESIAN_POINT('Ctrl Pts',(-4.632688642205,-42.6742356128,10.6483178932861));
#72064=CARTESIAN_POINT('Ctrl Pts',(-4.73537722156243,-42.6742356128,10.5130001325075));
#72065=CARTESIAN_POINT('Ctrl Pts',(-4.83785496840781,-42.6742356128,10.3779601960362));
#72066=CARTESIAN_POINT('Ctrl Pts',(-4.93455349622713,-42.6742356128,10.2385403525583));
#72067=CARTESIAN_POINT('Ctrl Pts',(-5.02511695345455,-42.6742356128,10.0952489230484));
#72068=CARTESIAN_POINT('Ctrl Pts',(-5.11539650363132,-42.6742356128,9.95240669731646));
#72069=CARTESIAN_POINT('Ctrl Pts',(-5.19957922013242,-42.6742356128,9.80571736998885));
#72070=CARTESIAN_POINT('Ctrl Pts',(-5.27735649408011,-42.6742356128,9.65571158802438));
#72071=CARTESIAN_POINT('Ctrl Pts',(-5.35478979332208,-42.6742356128,9.50636921571785));
#72072=CARTESIAN_POINT('Ctrl Pts',(-5.42587402836502,-42.6742356128,9.35373990520833));
#72073=CARTESIAN_POINT('Ctrl Pts',(-5.49035064036701,-42.6742356128,9.1983704838353));
#72074=CARTESIAN_POINT('Ctrl Pts',(-5.55446924847197,-42.6742356128,9.04386374517158));
#72075=CARTESIAN_POINT('Ctrl Pts',(-5.61205326919096,-42.6742356128,8.88664748173921));
#72076=CARTESIAN_POINT('Ctrl Pts',(-5.66289614742354,-42.6742356128,8.72727879847535));
#72077=CARTESIAN_POINT('Ctrl Pts',(-5.7132219012526,-42.6742356128,8.56953105875636));
#72078=CARTESIAN_POINT('Ctrl Pts',(-5.75694285303024,-42.6742356128,8.40967470181282));
#72079=CARTESIAN_POINT('Ctrl Pts',(-5.79390721110658,-42.6742356128,8.24826540145233));
#72080=CARTESIAN_POINT('Ctrl Pts',(-5.83063199617447,-42.6742356128,8.08790222535021));
#72081=CARTESIAN_POINT('Ctrl Pts',(-5.86068737210952,-42.6742356128,7.92600638961922));
#72082=CARTESIAN_POINT('Ctrl Pts',(-5.88397418321587,-42.6742356128,7.76313470857918));
#72083=CARTESIAN_POINT('Ctrl Pts',(-5.90700909826615,-42.6742356128,7.60202482884));
#72084=CARTESIAN_POINT('Ctrl Pts',(-5.92342102136939,-42.6742356128,7.43996031329963));
#72085=CARTESIAN_POINT('Ctrl Pts',(-5.93316405737334,-42.6742356128,7.27748855031532));
#72086=CARTESIAN_POINT('Ctrl Pts',(-5.93983232068902,-42.6742356128,7.16629071665196));
#72087=CARTESIAN_POINT('Ctrl Pts',(-5.94337776755146,-42.6742356128,7.05490229328725));
#72088=CARTESIAN_POINT('Ctrl Pts',(-5.94379970723532,-42.6742356128,6.94350032657215));
#72089=CARTESIAN_POINT('Ctrl Pts',(-5.9438282162108,-42.6742356128,6.93597328880065));
#72090=CARTESIAN_POINT('Ctrl Pts',(-5.94384245634447,-42.6742356128,6.9284462137));
#72091=CARTESIAN_POINT('Ctrl Pts',(-5.94384245598,-42.6742356128,6.92091847055));
#72092=CARTESIAN_POINT('',(-5.94384247076,-42.6742356128,3.43894174696));
#72093=CARTESIAN_POINT('',(-5.94384247076,-42.6742356128,1.43032185727));
#72094=CARTESIAN_POINT('',(-6.7528793859,-42.6742356128,2.63899279271));
#72095=CARTESIAN_POINT('Ctrl Pts',(-5.94384247076,-42.6742356128,3.43894174696));
#72096=CARTESIAN_POINT('Ctrl Pts',(-5.94384247076,-42.6742356128,3.39614059129875));
#72097=CARTESIAN_POINT('Ctrl Pts',(-5.94731942992889,-42.6742356127938,
3.3533935597809));
#72098=CARTESIAN_POINT('Ctrl Pts',(-5.95417334989511,-42.6742356127904,
3.31121746702997));
#72099=CARTESIAN_POINT('Ctrl Pts',(-5.95690615429115,-42.674235612789,3.29440095731788));
#72100=CARTESIAN_POINT('Ctrl Pts',(-5.96017526355245,-42.6742356127902,
3.27767531133813));
#72101=CARTESIAN_POINT('Ctrl Pts',(-5.96397199512074,-42.6742356127937,
3.26107340308066));
#72102=CARTESIAN_POINT('Ctrl Pts',(-5.97319230916015,-42.6742356128024,
3.22075588127698));
#72103=CARTESIAN_POINT('Ctrl Pts',(-5.98553169840033,-42.6742356128,3.1811674117174));
#72104=CARTESIAN_POINT('Ctrl Pts',(-6.00083792640887,-42.6742356128,3.14276485597422));
#72105=CARTESIAN_POINT('Ctrl Pts',(-6.00772218970423,-42.6742356128,3.12549258583667));
#72106=CARTESIAN_POINT('Ctrl Pts',(-6.0152059741815,-42.6742356128,3.10846008240039));
#72107=CARTESIAN_POINT('Ctrl Pts',(-6.02327205093866,-42.6742356128,3.09170791617586));
#72108=CARTESIAN_POINT('Ctrl Pts',(-6.03947059121232,-42.6742356128,3.05806570727695));
#72109=CARTESIAN_POINT('Ctrl Pts',(-6.05802013722139,-42.6742356128,3.02555577603168));
#72110=CARTESIAN_POINT('Ctrl Pts',(-6.07874913502031,-42.6742356128,2.99449840731163));
#72111=CARTESIAN_POINT('Ctrl Pts',(-6.09893208502231,-42.6742356128,2.96425915859585));
#72112=CARTESIAN_POINT('Ctrl Pts',(-6.12118191381689,-42.6742356128,2.93539676884652));
#72113=CARTESIAN_POINT('Ctrl Pts',(-6.14529655206815,-42.6742356128,2.90818632861611));
#72114=CARTESIAN_POINT('Ctrl Pts',(-6.16874740818222,-42.6742356128,2.88172488590256));
#72115=CARTESIAN_POINT('Ctrl Pts',(-6.19396202990645,-42.6742356128,2.85682550380557));
#72116=CARTESIAN_POINT('Ctrl Pts',(-6.22071762118132,-42.6742356128,2.83370869611102));
#72117=CARTESIAN_POINT('Ctrl Pts',(-6.22880357679397,-42.6742356128,2.82672243746309));
#72118=CARTESIAN_POINT('Ctrl Pts',(-6.2370299924312,-42.6742356128,2.81989877398227));
#72119=CARTESIAN_POINT('Ctrl Pts',(-6.24538996627878,-42.6742356128,2.8132432049317));
#72120=CARTESIAN_POINT('Ctrl Pts',(-6.27451151430862,-42.6742356128,2.79005886520695));
#72121=CARTESIAN_POINT('Ctrl Pts',(-6.30525732125456,-42.6742356128,2.76891658397484));
#72122=CARTESIAN_POINT('Ctrl Pts',(-6.33732192296069,-42.6742356127995,
2.75001660009913));
#72123=CARTESIAN_POINT('Ctrl Pts',(-6.35684144186036,-42.6742356127992,
2.73851112138318));
#72124=CARTESIAN_POINT('Ctrl Pts',(-6.37684937766888,-42.6742356127987,
2.72783553419962));
#72125=CARTESIAN_POINT('Ctrl Pts',(-6.39727405799141,-42.6742356127981,
2.71802609152613));
#72126=CARTESIAN_POINT('Ctrl Pts',(-6.43357980892323,-42.674235612797,2.70058938373633));
#72127=CARTESIAN_POINT('Ctrl Pts',(-6.47119967282077,-42.6742356127982,
2.68589341404767));
#72128=CARTESIAN_POINT('Ctrl Pts',(-6.50971611872968,-42.6742356127991,
2.67409624258505));
#72129=CARTESIAN_POINT('Ctrl Pts',(-6.5284451026621,-42.6742356127994,2.66835975705121));
#72130=CARTESIAN_POINT('Ctrl Pts',(-6.54738579197464,-42.6742356127997,
2.66330789205722));
#72131=CARTESIAN_POINT('Ctrl Pts',(-6.56648857804215,-42.6742356127998,
2.65895478335595));
#72132=CARTESIAN_POINT('Ctrl Pts',(-6.61310155549509,-42.6742356128001,
2.64833270147608));
#72133=CARTESIAN_POINT('Ctrl Pts',(-6.66068112877502,-42.6742356128,2.64187392258124));
#72134=CARTESIAN_POINT('Ctrl Pts',(-6.70850709539224,-42.6742356128,2.63973511372826));
#72135=CARTESIAN_POINT('Ctrl Pts',(-6.72065123224425,-42.6742356128,2.63919201989768));
#72136=CARTESIAN_POINT('Ctrl Pts',(-6.73281108748355,-42.6742356128,2.63892725618837));
#72137=CARTESIAN_POINT('Ctrl Pts',(-6.74497451472132,-42.6742356128,2.63894302968162));
#72138=CARTESIAN_POINT('Ctrl Pts',(-6.7476092010827,-42.6742356128,2.63894644633441));
#72139=CARTESIAN_POINT('Ctrl Pts',(-6.75024538341664,-42.6742356128,2.63896303862909));
#72140=CARTESIAN_POINT('Ctrl Pts',(-6.7528793859,-42.6742356128,2.63899279271));
#72141=CARTESIAN_POINT('',(-0.779583726501,-42.6742356128,-4.94563238948));
#72142=CARTESIAN_POINT('Ctrl Pts',(-6.7528793859,-42.6742356128,2.63899279271));
#72143=CARTESIAN_POINT('Ctrl Pts',(-6.92377102533431,-42.6742356128,2.64092304741057));
#72144=CARTESIAN_POINT('Ctrl Pts',(-7.09474113659899,-42.6742356128,2.63578350248769));
#72145=CARTESIAN_POINT('Ctrl Pts',(-7.26520473277953,-42.6742356128,2.62358798817555));
#72146=CARTESIAN_POINT('Ctrl Pts',(-7.43683936146178,-42.6742356128,2.61130869442924));
#72147=CARTESIAN_POINT('Ctrl Pts',(-7.60796025492586,-42.6742356128,2.59187623037914));
#72148=CARTESIAN_POINT('Ctrl Pts',(-7.77797524513836,-42.6742356128,2.56535760473604));
#72149=CARTESIAN_POINT('Ctrl Pts',(-7.94902508875408,-42.6742356128,2.53867756456142));
#72150=CARTESIAN_POINT('Ctrl Pts',(-8.11895527770663,-42.6742356128,2.50482492446711));
#72151=CARTESIAN_POINT('Ctrl Pts',(-8.28717142756282,-42.6742356128,2.46392001704393));
#72152=CARTESIAN_POINT('Ctrl Pts',(-8.45663566918383,-42.6742356128,2.42271161273214));
#72153=CARTESIAN_POINT('Ctrl Pts',(-8.62436007967723,-42.6742356128,2.37434598658467));
#72154=CARTESIAN_POINT('Ctrl Pts',(-8.78974957389737,-42.6742356128,2.31899759320297));
#72155=CARTESIAN_POINT('Ctrl Pts',(-8.95563157807734,-42.6742356128,2.26348437898347));
#72156=CARTESIAN_POINT('Ctrl Pts',(-9.11916447820672,-42.6742356128,2.20094687292207));
#72157=CARTESIAN_POINT('Ctrl Pts',(-9.27976444923896,-42.6742356128,2.13161100458411));
#72158=CARTESIAN_POINT('Ctrl Pts',(-9.44080179314795,-42.6742356128,2.06208630913739));
#72159=CARTESIAN_POINT('Ctrl Pts',(-9.59888994577529,-42.6742356128,1.98572630214571));
#72160=CARTESIAN_POINT('Ctrl Pts',(-9.75346091790575,-42.6742356128,1.90280695099595));
#72161=CARTESIAN_POINT('Ctrl Pts',(-9.85690152582706,-42.6742356128,1.84731640207106));
#72162=CARTESIAN_POINT('Ctrl Pts',(-9.95876741745598,-42.6742356128,1.78888928526941));
#72163=CARTESIAN_POINT('Ctrl Pts',(-10.0588943984393,-42.6742356128,1.72761986311077));
#72164=CARTESIAN_POINT('Ctrl Pts',(-10.2085963618408,-42.6742356128,1.63601465636686));
#72165=CARTESIAN_POINT('Ctrl Pts',(-10.3544080750074,-42.6742356128,1.53805489504499));
#72166=CARTESIAN_POINT('Ctrl Pts',(-10.4958044832224,-42.6742356128,1.43409260848261));
#72167=CARTESIAN_POINT('Ctrl Pts',(-10.6368847189839,-42.6742356128,1.3303627890078));
#72168=CARTESIAN_POINT('Ctrl Pts',(-10.7735691317831,-42.6742356128,1.22065742461589));
#72169=CARTESIAN_POINT('Ctrl Pts',(-10.9053668778309,-42.6742356128,1.10536790176509));
#72170=CARTESIAN_POINT('Ctrl Pts',(-11.0366971527523,-42.6742356128,0.990487297311773));
#72171=CARTESIAN_POINT('Ctrl Pts',(-11.1631751349909,-42.6742356128,0.870062247857544));
#72172=CARTESIAN_POINT('Ctrl Pts',(-11.2843492080509,-42.6742356128,0.744518921524571));
#72173=CARTESIAN_POINT('Ctrl Pts',(-11.4046009580189,-42.6742356128,0.619931175094103));
#72174=CARTESIAN_POINT('Ctrl Pts',(-11.5196290385353,-42.6742356128,0.490302959907881));
#72175=CARTESIAN_POINT('Ctrl Pts',(-11.6290287556409,-42.6742356128,0.356086480044981));
#72176=CARTESIAN_POINT('Ctrl Pts',(-11.7378494261036,-42.6742356128,0.222580400575742));
#72177=CARTESIAN_POINT('Ctrl Pts',(-11.8411009566513,-42.6742356128,0.0845346663024816));
#72178=CARTESIAN_POINT('Ctrl Pts',(-11.9384244464344,-42.6742356128,-0.0575728384140106));
#72179=CARTESIAN_POINT('Ctrl Pts',(-12.0348336088766,-42.6742356128,-0.198345282322419));
#72180=CARTESIAN_POINT('Ctrl Pts',(-12.1254254315195,-42.6742356128,-0.343103357163285));
#72181=CARTESIAN_POINT('Ctrl Pts',(-12.2098924354945,-42.6742356128,-0.491352838062098));
#72182=CARTESIAN_POINT('Ctrl Pts',(-12.268639735316,-42.6742356128,-0.594461227053108));
#72183=CARTESIAN_POINT('Ctrl Pts',(-12.3244251412665,-42.6742356128,-0.699257892387985));
#72184=CARTESIAN_POINT('Ctrl Pts',(-12.3771578279306,-42.6742356128,-0.805568642615839));
#72185=CARTESIAN_POINT('Ctrl Pts',(-12.4532257315113,-42.6742356128,-0.958923922035363));
#72186=CARTESIAN_POINT('Ctrl Pts',(-12.5229376336484,-42.6742356128,-1.11542736371576));
#72187=CARTESIAN_POINT('Ctrl Pts',(-12.5860515296792,-42.6742356128,-1.27454370014428));
#72188=CARTESIAN_POINT('Ctrl Pts',(-12.6496267367883,-42.6742356128,-1.43482304715101));
#72189=CARTESIAN_POINT('Ctrl Pts',(-12.7065070981696,-42.6742356128,-1.597753382621));
#72190=CARTESIAN_POINT('Ctrl Pts',(-12.7564952320637,-42.6742356128,-1.76276934411767));
#72191=CARTESIAN_POINT('Ctrl Pts',(-12.8068026288887,-42.6742356128,-1.92883922532304));
#72192=CARTESIAN_POINT('Ctrl Pts',(-12.8501294506246,-42.6742356128,-2.09702120108295));
#72193=CARTESIAN_POINT('Ctrl Pts',(-12.8863254015399,-42.6742356128,-2.26672434958655));
#72194=CARTESIAN_POINT('Ctrl Pts',(-12.9227119363533,-42.6742356128,-2.43732104244341));
#72195=CARTESIAN_POINT('Ctrl Pts',(-12.9518922903244,-42.6742356128,-2.60945469813757));
#72196=CARTESIAN_POINT('Ctrl Pts',(-12.9737653933523,-42.6742356128,-2.78251424103995));
#72197=CARTESIAN_POINT('Ctrl Pts',(-12.9957250456641,-42.6742356128,-2.95625856010277));
#72198=CARTESIAN_POINT('Ctrl Pts',(-13.0103194960362,-42.6742356128,-3.13093582595532));
#72199=CARTESIAN_POINT('Ctrl Pts',(-13.0174985506679,-42.6742356128,-3.30592102821733));
#72200=CARTESIAN_POINT('Ctrl Pts',(-13.0249406122865,-42.6742356128,-3.48731686992664));
#72201=CARTESIAN_POINT('Ctrl Pts',(-13.0244136769526,-42.6742356128,-3.66904331228793));
#72202=CARTESIAN_POINT('Ctrl Pts',(-13.0159205917797,-42.6742356128,-3.85040149710429));
#72203=CARTESIAN_POINT('Ctrl Pts',(-13.0077589161263,-42.6742356128,-4.02468288619295));
#72204=CARTESIAN_POINT('Ctrl Pts',(-12.9922406788355,-42.6742356128,-4.19862603527503));
#72205=CARTESIAN_POINT('Ctrl Pts',(-12.9694214754203,-42.6742356128,-4.37160392560452));
#72206=CARTESIAN_POINT('Ctrl Pts',(-12.9464802820924,-42.6742356128,-4.54550654399528));
#72207=CARTESIAN_POINT('Ctrl Pts',(-12.9161600388264,-42.6742356128,-4.71843359904739));
#72208=CARTESIAN_POINT('Ctrl Pts',(-12.8785687783075,-42.6742356128,-4.8897636315973));
#72209=CARTESIAN_POINT('Ctrl Pts',(-12.8410768237495,-42.6742356128,-5.06064105645925));
#72210=CARTESIAN_POINT('Ctrl Pts',(-12.7963522654434,-42.6742356128,-5.2299296012495));
#72211=CARTESIAN_POINT('Ctrl Pts',(-12.7445528469835,-42.6742356128,-5.39702377187447));
#72212=CARTESIAN_POINT('Ctrl Pts',(-12.692955085043,-42.6742356128,-5.56346744043058));
#72213=CARTESIAN_POINT('Ctrl Pts',(-12.6343374980566,-42.6742356128,-5.72773351285106));
#72214=CARTESIAN_POINT('Ctrl Pts',(-12.5689054311692,-42.6742356128,-5.88923868726432));
#72215=CARTESIAN_POINT('Ctrl Pts',(-12.5039776015438,-42.6742356128,-6.04949925898035));
#72216=CARTESIAN_POINT('Ctrl Pts',(-12.4323400011397,-42.6742356128,-6.20704107056944));
#72217=CARTESIAN_POINT('Ctrl Pts',(-12.3542409292231,-42.6742356128,-6.36131303593145));
#72218=CARTESIAN_POINT('Ctrl Pts',(-12.2765647547587,-42.6742356128,-6.51474963642295));
#72219=CARTESIAN_POINT('Ctrl Pts',(-12.1924969600612,-42.6742356128,-6.66495145996804));
#72220=CARTESIAN_POINT('Ctrl Pts',(-12.1023280783887,-42.6742356128,-6.81139873697023));
#72221=CARTESIAN_POINT('Ctrl Pts',(-12.0129470463386,-42.6742356128,-6.95656643248342));
#72222=CARTESIAN_POINT('Ctrl Pts',(-11.9175711644125,-42.6742356128,-7.09804468603061));
#72223=CARTESIAN_POINT('Ctrl Pts',(-11.8165278203223,-42.6742356128,-7.23535275773844));
#72224=CARTESIAN_POINT('Ctrl Pts',(-11.7830752393437,-42.6742356128,-7.28081155989094));
#72225=CARTESIAN_POINT('Ctrl Pts',(-11.7490018150758,-42.6742356128,-7.32581349837004));
#72226=CARTESIAN_POINT('Ctrl Pts',(-11.7143204894683,-42.6742356128,-7.37034181538974));
#72227=CARTESIAN_POINT('Ctrl Pts',(-11.6090374799616,-42.6742356128,-7.50551759491913));
#72228=CARTESIAN_POINT('Ctrl Pts',(-11.4981515428722,-42.6742356128,-7.63632322849263));
#72229=CARTESIAN_POINT('Ctrl Pts',(-11.3820409767117,-42.6742356128,-7.76230784158382));
#72230=CARTESIAN_POINT('Ctrl Pts',(-11.2650896267103,-42.6742356128,-7.88920473880554));
#72231=CARTESIAN_POINT('Ctrl Pts',(-11.1428379117467,-42.6742356128,-8.01121040408434));
#72232=CARTESIAN_POINT('Ctrl Pts',(-11.0157106099601,-42.6742356128,-8.12790111131797));
#72233=CARTESIAN_POINT('Ctrl Pts',(-10.8877834955309,-42.6742356128,-8.24532597008016));
#72234=CARTESIAN_POINT('Ctrl Pts',(-10.7549194727002,-42.6742356128,-8.35736864419994));
#72235=CARTESIAN_POINT('Ctrl Pts',(-10.6175867190644,-42.6742356128,-8.46363679340583));
#72236=CARTESIAN_POINT('Ctrl Pts',(-10.4795477508587,-42.6742356128,-8.57045141177738));
#72237=CARTESIAN_POINT('Ctrl Pts',(-10.3369942102914,-42.6742356128,-8.67143182642991));
#72238=CARTESIAN_POINT('Ctrl Pts',(-10.1904336618126,-42.6742356128,-8.76622139845801));
#72239=CARTESIAN_POINT('Ctrl Pts',(-10.0433150051289,-42.6742356128,-8.86137193282168));
#72240=CARTESIAN_POINT('Ctrl Pts',(-9.89215901548288,-42.6742356128,-8.95028425309374));
#72241=CARTESIAN_POINT('Ctrl Pts',(-9.73750768486439,-42.6742356128,-9.03264163716008));
#72242=CARTESIAN_POINT('Ctrl Pts',(-9.57733278527883,-42.6742356128,-9.11794051994497));
#72243=CARTESIAN_POINT('Ctrl Pts',(-9.41340855055791,-42.6742356128,-9.19620745294721));
#72244=CARTESIAN_POINT('Ctrl Pts',(-9.24636493029186,-42.6742356128,-9.26714220767078));
#72245=CARTESIAN_POINT('Ctrl Pts',(-9.10197090675754,-42.6742356128,-9.32845885434453));
#72246=CARTESIAN_POINT('Ctrl Pts',(-8.95524480384927,-42.6742356128,-9.38429823234259));
#72247=CARTESIAN_POINT('Ctrl Pts',(-8.80661470177786,-42.6742356128,-9.43449693353395));
#72248=CARTESIAN_POINT('Ctrl Pts',(-8.64045654990412,-42.6742356128,-9.49061560196096));
#72249=CARTESIAN_POINT('Ctrl Pts',(-8.47191949133974,-42.6742356128,-9.5396838161239));
#72250=CARTESIAN_POINT('Ctrl Pts',(-8.30160860483715,-42.6742356128,-9.5815245018864));
#72251=CARTESIAN_POINT('Ctrl Pts',(-8.13175340326074,-42.6742356128,-9.62325323843535));
#72252=CARTESIAN_POINT('Ctrl Pts',(-7.960134129673,-42.6742356128,-9.65779298871373));
#72253=CARTESIAN_POINT('Ctrl Pts',(-7.78736340133293,-42.6742356128,-9.68501834033365));
#72254=CARTESIAN_POINT('Ctrl Pts',(-7.61527114017249,-42.6742356128,-9.71213677854465));
#72255=CARTESIAN_POINT('Ctrl Pts',(-7.44203672137731,-42.6742356128,-9.7319980826045));
#72256=CARTESIAN_POINT('Ctrl Pts',(-7.26827378018691,-42.6742356128,-9.74452934705639));
#72257=CARTESIAN_POINT('Ctrl Pts',(-7.09587297012232,-42.6742356128,-9.7569623786789));
#72258=CARTESIAN_POINT('Ctrl Pts',(-6.92295215394564,-42.6742356128,-9.76217980786957));
#72259=CARTESIAN_POINT('Ctrl Pts',(-6.75011476368856,-42.6742356128,-9.7601614805935));
#72260=CARTESIAN_POINT('Ctrl Pts',(-6.57821936998901,-42.6742356128,-9.75815415358388));
#72261=CARTESIAN_POINT('Ctrl Pts',(-6.40640674483326,-42.6742356128,-9.74898967690743));
#72262=CARTESIAN_POINT('Ctrl Pts',(-6.2352707865071,-42.6742356128,-9.73269957300655));
#72263=CARTESIAN_POINT('Ctrl Pts',(-6.06567484140039,-42.6742356128,-9.71655606001268));
#72264=CARTESIAN_POINT('Ctrl Pts',(-5.89674367410256,-42.6742356128,-9.69341456947751));
#72265=CARTESIAN_POINT('Ctrl Pts',(-5.72905197408973,-42.6742356128,-9.66335680406608));
#72266=CARTESIAN_POINT('Ctrl Pts',(-5.65633979088631,-42.6742356128,-9.65032356661238));
#72267=CARTESIAN_POINT('Ctrl Pts',(-5.58386058221207,-42.6742356128,-9.63599062406029));
#72268=CARTESIAN_POINT('Ctrl Pts',(-5.51166083356658,-42.6742356128,-9.62036767336498));
#72269=CARTESIAN_POINT('Ctrl Pts',(-5.34553008021385,-42.6742356128,-9.58441945169806));
#72270=CARTESIAN_POINT('Ctrl Pts',(-5.18088487182742,-42.6742356128,-9.54163888505871));
#72271=CARTESIAN_POINT('Ctrl Pts',(-5.01828069868697,-42.6742356128,-9.49216531343611));
#72272=CARTESIAN_POINT('Ctrl Pts',(-4.85368753416137,-42.6742356128,-9.44208657587067));
#72273=CARTESIAN_POINT('Ctrl Pts',(-4.69118586381926,-42.6742356128,-9.38515019160763));
#72274=CARTESIAN_POINT('Ctrl Pts',(-4.53133558518016,-42.6742356127989,
-9.32155164731861));
#72275=CARTESIAN_POINT('Ctrl Pts',(-4.37049551713942,-42.6742356127977,
-9.25755930224529));
#72276=CARTESIAN_POINT('Ctrl Pts',(-4.21233999388847,-42.6742356127957,
-9.18682219542086));
#72277=CARTESIAN_POINT('Ctrl Pts',(-4.05741975468309,-42.6742356127869,
-9.10958874043621));
#72278=CARTESIAN_POINT('Ctrl Pts',(-3.9012794912673,-42.674235612778,-9.03174705837019));
#72279=CARTESIAN_POINT('Ctrl Pts',(-3.74842590424833,-42.6742356127626,
-8.94730645802646));
#72280=CARTESIAN_POINT('Ctrl Pts',(-3.59939955038934,-42.6742356127243,
-8.85656883986676));
#72281=CARTESIAN_POINT('Ctrl Pts',(-3.52827949945173,-42.6742356127061,
-8.81326600209095));
#72282=CARTESIAN_POINT('Ctrl Pts',(-3.45803073797694,-42.6742356126824,
-8.76852969966192));
#72283=CARTESIAN_POINT('Ctrl Pts',(-3.38870993135324,-42.67423561265,-8.7223963607209));
#72284=CARTESIAN_POINT('Ctrl Pts',(-3.24323874551504,-42.6742356125822,
-8.62558456857231));
#72285=CARTESIAN_POINT('Ctrl Pts',(-3.10185699243564,-42.6742356125117,
-8.52261712902016));
#72286=CARTESIAN_POINT('Ctrl Pts',(-2.96506951706885,-42.6742356124598,
-8.41386451273636));
#72287=CARTESIAN_POINT('Ctrl Pts',(-2.82781328827125,-42.6742356124077,
-8.30473921494896));
#72288=CARTESIAN_POINT('Ctrl Pts',(-2.69518312142502,-42.6742356123738,
-8.18978922737835));
#72289=CARTESIAN_POINT('Ctrl Pts',(-2.56765662468396,-42.6742356123612,
-8.06943004369615));
#72290=CARTESIAN_POINT('Ctrl Pts',(-2.44012637314771,-42.6742356123487,
-7.94906731624778));
#72291=CARTESIAN_POINT('Ctrl Pts',(-2.31770031683979,-42.6742356123569,
-7.82329530435268));
#72292=CARTESIAN_POINT('Ctrl Pts',(-2.20082023554204,-42.6742356123795,
-7.69256736730877));
#72293=CARTESIAN_POINT('Ctrl Pts',(-2.08412128240898,-42.674235612402,-7.5620420183453));
#72294=CARTESIAN_POINT('Ctrl Pts',(-1.97295134094947,-42.6742356124384,
-7.42657633123456));
#72295=CARTESIAN_POINT('Ctrl Pts',(-1.86771112173087,-42.6742356124791,
-7.28665574540306));
#72296=CARTESIAN_POINT('Ctrl Pts',(-1.76279308389599,-42.6742356125197,
-7.14716351109238));
#72297=CARTESIAN_POINT('Ctrl Pts',(-1.6637687149937,-42.6742356125643,-7.00324385547099));
#72298=CARTESIAN_POINT('Ctrl Pts',(-1.57099319647258,-42.6742356126051,
-6.85540816315929));
#72299=CARTESIAN_POINT('Ctrl Pts',(-1.47891116550525,-42.6742356126455,
-6.7086775275938));
#72300=CARTESIAN_POINT('Ctrl Pts',(-1.39298507142996,-42.674235612682,-6.55808943413321));
#72301=CARTESIAN_POINT('Ctrl Pts',(-1.31351830313044,-42.6742356127107,
-6.40417013889175));
#72302=CARTESIAN_POINT('Ctrl Pts',(-1.23447264371694,-42.6742356127392,
-6.25106649004366));
#72303=CARTESIAN_POINT('Ctrl Pts',(-1.16181819676399,-42.67423561276,-6.09466708554217));
#72304=CARTESIAN_POINT('Ctrl Pts',(-1.09580756166894,-42.6742356127736,
-5.9355123158406));
#72305=CARTESIAN_POINT('Ctrl Pts',(-1.0304709446788,-42.6742356127871,-5.77798263573418));
#72306=CARTESIAN_POINT('Ctrl Pts',(-0.971643269281571,-42.6742356127937,
-5.61775380907576));
#72307=CARTESIAN_POINT('Ctrl Pts',(-0.919522300230464,-42.6742356127969,
-5.45536837298743));
#72308=CARTESIAN_POINT('Ctrl Pts',(-0.867847187573667,-42.6742356128,-5.29437202436889));
#72309=CARTESIAN_POINT('Ctrl Pts',(-0.822764645901731,-42.6742356128,-5.13125602266412));
#72310=CARTESIAN_POINT('Ctrl Pts',(-0.78441907782484,-42.6742356128,-4.96656404596631));
#72311=CARTESIAN_POINT('Ctrl Pts',(-0.782795283673876,-42.6742356128,-4.95958994486716));
#72312=CARTESIAN_POINT('Ctrl Pts',(-0.781183576258786,-42.6742356128,-4.95261299441384));
#72313=CARTESIAN_POINT('Ctrl Pts',(-0.779583726501,-42.6742356128,-4.94563238948));
#72314=CARTESIAN_POINT('',(-1.92001921505849E-7,-42.6742356128,-4.32434669440466));
#72315=CARTESIAN_POINT('Ctrl Pts',(-0.779583726501,-42.6742356128,-4.94563238948));
#72316=CARTESIAN_POINT('Ctrl Pts',(-0.770339586016146,-42.6742356128,-4.90529749155185));
#72317=CARTESIAN_POINT('Ctrl Pts',(-0.757952557321631,-42.6742356128,-4.86571925121627));
#72318=CARTESIAN_POINT('Ctrl Pts',(-0.742592335257283,-42.6742356128,-4.82734087116641));
#72319=CARTESIAN_POINT('Ctrl Pts',(-0.727732731079844,-42.6742356128,-4.79021331310618));
#72320=CARTESIAN_POINT('Ctrl Pts',(-0.71009068241812,-42.6742356128,-4.75420963049573));
#72321=CARTESIAN_POINT('Ctrl Pts',(-0.689867037474384,-42.6742356128,-4.71972195099769));
#72322=CARTESIAN_POINT('Ctrl Pts',(-0.67972492593344,-42.6742356128,-4.7024264588532));
#72323=CARTESIAN_POINT('Ctrl Pts',(-0.668934286154698,-42.6742356128,-4.6855120087769));
#72324=CARTESIAN_POINT('Ctrl Pts',(-0.657525035376213,-42.6742356128,-4.66902604106184));
#72325=CARTESIAN_POINT('Ctrl Pts',(-0.636024130235446,-42.6742356128,-4.63795798629844));
#72326=CARTESIAN_POINT('Ctrl Pts',(-0.612323425048321,-42.6742356128,-4.60841296301403));
#72327=CARTESIAN_POINT('Ctrl Pts',(-0.586653996613761,-42.6742356128,-4.5806891190954));
#72328=CARTESIAN_POINT('Ctrl Pts',(-0.577855991671729,-42.6742356128,-4.57118697858495));
#72329=CARTESIAN_POINT('Ctrl Pts',(-0.568827070431133,-42.6742356128,-4.56189851480791));
#72330=CARTESIAN_POINT('Ctrl Pts',(-0.559577658427724,-42.6742356128,-4.55283483251327));
#72331=CARTESIAN_POINT('Ctrl Pts',(-0.53393557106704,-42.6742356128,-4.52770764246886));
#72332=CARTESIAN_POINT('Ctrl Pts',(-0.506597397053191,-42.6742356128,-4.50431172009628));
#72333=CARTESIAN_POINT('Ctrl Pts',(-0.477809692424286,-42.6742356128,-4.48286055934883));
#72334=CARTESIAN_POINT('Ctrl Pts',(-0.465912990238111,-42.6742356128,-4.47399573062247));
#72335=CARTESIAN_POINT('Ctrl Pts',(-0.453769151708002,-42.6742356128,-4.46546260164222));
#72336=CARTESIAN_POINT('Ctrl Pts',(-0.44139735549178,-42.6742356128,-4.45727428681099));
#72337=CARTESIAN_POINT('Ctrl Pts',(-0.410257347175726,-42.6742356128,-4.43666416783696));
#72338=CARTESIAN_POINT('Ctrl Pts',(-0.377671015886976,-42.6742356128001,
-4.41824161902664));
#72339=CARTESIAN_POINT('Ctrl Pts',(-0.343960679444774,-42.6742356127991,
-4.40218302518042));
#72340=CARTESIAN_POINT('Ctrl Pts',(-0.331872099374508,-42.6742356127987,
-4.39642438797848));
#72341=CARTESIAN_POINT('Ctrl Pts',(-0.319639082799004,-42.6742356127982,
-4.39096925555829));
#72342=CARTESIAN_POINT('Ctrl Pts',(-0.30727685469933,-42.6742356127976,
-4.3858242042423));
#72343=CARTESIAN_POINT('Ctrl Pts',(-0.270146176475813,-42.6742356127959,
-4.37037074040737));
#72344=CARTESIAN_POINT('Ctrl Pts',(-0.23185666760706,-42.6742356127962,
-4.35772125484493));
#72345=CARTESIAN_POINT('Ctrl Pts',(-0.192827890891106,-42.6742356127974,
-4.3480119902983));
#72346=CARTESIAN_POINT('Ctrl Pts',(-0.151055129146623,-42.6742356127986,
-4.33762009926949));
#72347=CARTESIAN_POINT('Ctrl Pts',(-0.108435042767796,-42.6742356127998,
-4.33059591170187));
#72348=CARTESIAN_POINT('Ctrl Pts',(-0.0655037400434273,-42.6742356127999,
-4.32705002118447));
#72349=CARTESIAN_POINT('Ctrl Pts',(-0.0473517386002392,-42.6742356128,-4.32555076526385));
#72350=CARTESIAN_POINT('Ctrl Pts',(-0.0291443943596306,-42.6742356128,-4.32467272136695));
#72351=CARTESIAN_POINT('Ctrl Pts',(-0.0109235923233173,-42.6742356128,-4.32442189871929));
#72352=CARTESIAN_POINT('Ctrl Pts',(-0.0072829618668721,-42.6742356128,-4.32437178278211));
#72353=CARTESIAN_POINT('Ctrl Pts',(-0.00364100425362554,-42.6742356128,
-4.32434670023877));
#72354=CARTESIAN_POINT('Ctrl Pts',(-3.83477804066779E-7,-42.6742356128,
-4.32434669416));
#72355=CARTESIAN_POINT('Ctrl Pts',(-6.27276008913E-15,-42.6742356128,-4.32434669465));
#72356=CARTESIAN_POINT('Ctrl Pts',(0.0418710994610801,-42.6742356128,-4.32434671500355));
#72357=CARTESIAN_POINT('Ctrl Pts',(0.0837043788816997,-42.6742356128,-4.3276623402763));
#72358=CARTESIAN_POINT('Ctrl Pts',(0.125013272835771,-42.6742356128,-4.33422057793384));
#72359=CARTESIAN_POINT('Ctrl Pts',(0.164771346375193,-42.6742356128,-4.34053260592876));
#72360=CARTESIAN_POINT('Ctrl Pts',(0.204042705126419,-42.6742356128,-4.34984847391554));
#72361=CARTESIAN_POINT('Ctrl Pts',(0.242392380067074,-42.6742356128,-4.362055492168));
#72362=CARTESIAN_POINT('Ctrl Pts',(0.260743896289878,-42.6742356128,-4.36789693134157));
#72363=CARTESIAN_POINT('Ctrl Pts',(0.278884424047291,-42.6742356128,-4.37439969445921));
#72364=CARTESIAN_POINT('Ctrl Pts',(0.296767143629254,-42.6742356128,-4.38154722137599));
#72365=CARTESIAN_POINT('Ctrl Pts',(0.331742254434663,-42.6742356128,-4.39552638963131));
#72366=CARTESIAN_POINT('Ctrl Pts',(0.365730473692324,-42.6742356128,-4.4119749533356));
#72367=CARTESIAN_POINT('Ctrl Pts',(0.39839280384516,-42.6742356128,-4.43073575255324));
#72368=CARTESIAN_POINT('Ctrl Pts',(0.429691506349557,-42.6742356128,-4.44871330255381));
#72369=CARTESIAN_POINT('Ctrl Pts',(0.459772353724042,-42.6742356128,-4.46881415672584));
#72370=CARTESIAN_POINT('Ctrl Pts',(0.48835644570818,-42.6742356128,-4.49085721429512));
#72371=CARTESIAN_POINT('Ctrl Pts',(0.510283685623865,-42.6742356128,-4.50776673907783));
#72372=CARTESIAN_POINT('Ctrl Pts',(0.531330750563295,-42.6742356128,-4.52581851907484));
#72373=CARTESIAN_POINT('Ctrl Pts',(0.551383898576014,-42.6742356128,-4.54491381005563));
#72374=CARTESIAN_POINT('Ctrl Pts',(0.578386538937482,-42.6742356128,-4.57062664450061));
#72375=CARTESIAN_POINT('Ctrl Pts',(0.603585765744263,-42.6742356128001,
-4.59823263562595));
#72376=CARTESIAN_POINT('Ctrl Pts',(0.62673854776236,-42.6742356127992,-4.62745825901451));
#72377=CARTESIAN_POINT('Ctrl Pts',(0.635091421482877,-42.6742356127989,
-4.63800204340195));
#72378=CARTESIAN_POINT('Ctrl Pts',(0.643178393391744,-42.6742356127985,
-4.64875641850709));
#72379=CARTESIAN_POINT('Ctrl Pts',(0.650989517822355,-42.674235612798,-4.65970782242662));
#72380=CARTESIAN_POINT('Ctrl Pts',(0.674231624148513,-42.6742356127964,
-4.69229387281917));
#72381=CARTESIAN_POINT('Ctrl Pts',(0.695023442466847,-42.6742356127966,
-4.72661905129764));
#72382=CARTESIAN_POINT('Ctrl Pts',(0.713142368797677,-42.6742356127976,
-4.76230994089147));
#72383=CARTESIAN_POINT('Ctrl Pts',(0.732451655575785,-42.6742356127987,
-4.80034561750661));
#72384=CARTESIAN_POINT('Ctrl Pts',(0.748725829968211,-42.6742356127998,
-4.83993264972833));
#72385=CARTESIAN_POINT('Ctrl Pts',(0.761745590136327,-42.6742356127999,
-4.88058615396062));
#72386=CARTESIAN_POINT('Ctrl Pts',(0.767488735920299,-42.6742356128,-4.89851881926478));
#72387=CARTESIAN_POINT('Ctrl Pts',(0.772599221477852,-42.6742356128,-4.91665855611848));
#72388=CARTESIAN_POINT('Ctrl Pts',(0.777060571531673,-42.6742356128,-4.93496167066254));
#72389=CARTESIAN_POINT('Ctrl Pts',(0.777815731721221,-42.6742356128,-4.93805978743923));
#72390=CARTESIAN_POINT('Ctrl Pts',(0.778552314305808,-42.6742356128,-4.94116264967606));
#72391=CARTESIAN_POINT('Ctrl Pts',(0.779270224014823,-42.6742356128,-4.94426996798293));
#72392=CARTESIAN_POINT('Ctrl Pts',(0.779375237689296,-42.6742356128,-4.94472449716545));
#72393=CARTESIAN_POINT('Ctrl Pts',(0.779479851147667,-42.6742356128,-4.94517911900667));
#72394=CARTESIAN_POINT('Ctrl Pts',(0.779584041801,-42.6742356128,-4.94563373444));
#72395=CARTESIAN_POINT('',(5.54384247000667,-42.6742356128,3.12351053169));
#72396=CARTESIAN_POINT('',(5.54384245881164,-42.6742356128,6.92091963994));
#72397=CARTESIAN_POINT('',(5.54384247076,-42.6742356128,1.77756718468));
#72398=CARTESIAN_POINT('',(4.98144931501833,-42.6742356128,2.35961165425857));
#72399=CARTESIAN_POINT('Ctrl Pts',(4.98144948316736,-42.6742356128,2.35961170656036));
#72400=CARTESIAN_POINT('Ctrl Pts',(5.02061454614235,-42.6742356128,2.37179381057219));
#72401=CARTESIAN_POINT('Ctrl Pts',(5.05880901067664,-42.6742356128,2.38699634304257));
#72402=CARTESIAN_POINT('Ctrl Pts',(5.0956106138185,-42.6742356128,2.40502524049932));
#72403=CARTESIAN_POINT('Ctrl Pts',(5.13126969987241,-42.6742356128,2.4224944252897));
#72404=CARTESIAN_POINT('Ctrl Pts',(5.16562018730549,-42.6742356128,2.44261704816507));
#72405=CARTESIAN_POINT('Ctrl Pts',(5.19829190310246,-42.6742356128,2.4651700559157));
#72406=CARTESIAN_POINT('Ctrl Pts',(5.21049951593566,-42.6742356128,2.47359686730678));
#72407=CARTESIAN_POINT('Ctrl Pts',(5.22247296352245,-42.6742356128,2.48236252078492));
#72408=CARTESIAN_POINT('Ctrl Pts',(5.23419382990894,-42.6742356128,2.49145370342273));
#72409=CARTESIAN_POINT('Ctrl Pts',(5.26403643920578,-42.6742356128,2.51460084993566));
#72410=CARTESIAN_POINT('Ctrl Pts',(5.29223950540321,-42.6742356128,2.53986119092365));
#72411=CARTESIAN_POINT('Ctrl Pts',(5.31851865739924,-42.6742356128,2.5669873519108));
#72412=CARTESIAN_POINT('Ctrl Pts',(5.32550593200998,-42.6742356128,2.57419983486996));
#72413=CARTESIAN_POINT('Ctrl Pts',(5.33235737434974,-42.6742356128,2.58154400578135));
#72414=CARTESIAN_POINT('Ctrl Pts',(5.33906805847429,-42.6742356128,2.58901473966406));
#72415=CARTESIAN_POINT('Ctrl Pts',(5.36318747049904,-42.6742356128,2.61586590793544));
#72416=CARTESIAN_POINT('Ctrl Pts',(5.38548485109696,-42.6742356128,2.64435374065739));
#72417=CARTESIAN_POINT('Ctrl Pts',(5.40575467525082,-42.6742356128,2.67421842643644));
#72418=CARTESIAN_POINT('Ctrl Pts',(5.41233781008693,-42.6742356128,2.6839177337333));
#72419=CARTESIAN_POINT('Ctrl Pts',(5.41870738243033,-42.6742356128,2.69376200286744));
#72420=CARTESIAN_POINT('Ctrl Pts',(5.42485727315772,-42.6742356128,2.70374155831051));
#72421=CARTESIAN_POINT('Ctrl Pts',(5.4444023437645,-42.6742356128,2.73545775041947));
#72422=CARTESIAN_POINT('Ctrl Pts',(5.46172526525044,-42.6742356128,2.76854259355569));
#72423=CARTESIAN_POINT('Ctrl Pts',(5.4766603444294,-42.6742356127988,2.80266885969859));
#72424=CARTESIAN_POINT('Ctrl Pts',(5.49214926650727,-42.6742356127975,2.83806064241109));
#72425=CARTESIAN_POINT('Ctrl Pts',(5.50507023096377,-42.674235612795,2.87457310110306));
#72426=CARTESIAN_POINT('Ctrl Pts',(5.51529386257496,-42.6742356127955,2.91183085727209));
#72427=CARTESIAN_POINT('Ctrl Pts',(5.52051739832013,-42.6742356127958,2.93086687387907));
#72428=CARTESIAN_POINT('Ctrl Pts',(5.52503765376591,-42.674235612797,2.95009722852049));
#72429=CARTESIAN_POINT('Ctrl Pts',(5.52884225515805,-42.6742356127983,2.96947009082168));
#72430=CARTESIAN_POINT('Ctrl Pts',(5.53697901810226,-42.6742356128011,3.01090212846463));
#72431=CARTESIAN_POINT('Ctrl Pts',(5.54183789209737,-42.6742356128,3.05298314735757));
#72432=CARTESIAN_POINT('Ctrl Pts',(5.54333924500842,-42.6742356128,3.09520879650193));
#72433=CARTESIAN_POINT('Ctrl Pts',(5.54364552076626,-42.6742356128,3.10382282228966));
#72434=CARTESIAN_POINT('Ctrl Pts',(5.54381218081857,-42.6742356128,3.11244273439275));
#72435=CARTESIAN_POINT('Ctrl Pts',(5.54383870476508,-42.6742356128,3.12106402816618));
#72436=CARTESIAN_POINT('Ctrl Pts',(5.54384121393877,-42.6742356128,3.12187960527063));
#72437=CARTESIAN_POINT('Ctrl Pts',(5.54384246876333,-42.6742356128,3.12269520399));
#72438=CARTESIAN_POINT('Ctrl Pts',(5.54384246963,-42.6742356128,3.12351053169));
#72439=CARTESIAN_POINT('',(0.7797602054102,-42.6742356128,-2.1748213248982));
#72440=CARTESIAN_POINT('Ctrl Pts',(0.779760433538598,-42.6742356128,-2.17482033007699));
#72441=CARTESIAN_POINT('Ctrl Pts',(0.82008088638103,-42.6742356128,-1.99899136424202));
#72442=CARTESIAN_POINT('Ctrl Pts',(0.868120974796676,-42.6742356128,-1.82488581137916));
#72443=CARTESIAN_POINT('Ctrl Pts',(0.923660857455244,-42.6742356128,-1.65320006696145));
#72444=CARTESIAN_POINT('Ctrl Pts',(0.978754958155079,-42.6742356128,-1.48289233063035));
#72445=CARTESIAN_POINT('Ctrl Pts',(1.04122908190946,-42.6742356128,-1.31496565181674));
#72446=CARTESIAN_POINT('Ctrl Pts',(1.11083180500875,-42.6742356128,-1.15006455618185));
#72447=CARTESIAN_POINT('Ctrl Pts',(1.17987810904471,-42.6742356128,-0.986481715194041));
#72448=CARTESIAN_POINT('Ctrl Pts',(1.25593962112789,-42.6742356128,-0.825876216584327));
#72449=CARTESIAN_POINT('Ctrl Pts',(1.33873253370372,-42.6742356128,-0.668843344668419));
#72450=CARTESIAN_POINT('Ctrl Pts',(1.42051548793609,-42.6742356128,-0.513726055309701));
#72451=CARTESIAN_POINT('Ctrl Pts',(1.50886670645572,-42.6742356128,-0.36209468242655));
#72452=CARTESIAN_POINT('Ctrl Pts',(1.60347348717891,-42.6742356128,-0.214490841091055));
#72453=CARTESIAN_POINT('Ctrl Pts',(1.69744929431954,-42.6742356128,-0.067871433681505));
#72454=CARTESIAN_POINT('Ctrl Pts',(1.79759761771214,-42.6742356128,0.0747740334099692));
#72455=CARTESIAN_POINT('Ctrl Pts',(1.90357150485393,-42.6742356128,0.212945727140077));
#72456=CARTESIAN_POINT('Ctrl Pts',(2.00841817475825,-42.6742356128,0.349647723767401));
#72457=CARTESIAN_POINT('Ctrl Pts',(2.11896721928139,-42.6742356128,0.481970679030743));
#72458=CARTESIAN_POINT('Ctrl Pts',(2.23484145936028,-42.6742356128,0.609460133745291));
#72459=CARTESIAN_POINT('Ctrl Pts',(2.33817498809426,-42.6742356128,0.723151798286571));
#72460=CARTESIAN_POINT('Ctrl Pts',(2.445742944833,-42.6742356128,0.832999982031719));
#72461=CARTESIAN_POINT('Ctrl Pts',(2.55724886492688,-42.6742356128,0.938702013268061));
#72462=CARTESIAN_POINT('Ctrl Pts',(2.68199902176198,-42.6742356128,1.05695891804424));
#72463=CARTESIAN_POINT('Ctrl Pts',(2.81167944725901,-42.6742356128,1.17002607613155));
#72464=CARTESIAN_POINT('Ctrl Pts',(2.94584550454677,-42.6742356128,1.27751782547255));
#72465=CARTESIAN_POINT('Ctrl Pts',(3.08194386060407,-42.6742356128,1.38655770240398));
#72466=CARTESIAN_POINT('Ctrl Pts',(3.22265784039016,-42.6742356128,1.48986042507482));
#72467=CARTESIAN_POINT('Ctrl Pts',(3.36748660588292,-42.6742356128,1.58706255794715));
#72468=CARTESIAN_POINT('Ctrl Pts',(3.51565498560908,-42.6742356128,1.68650607998932));
#72469=CARTESIAN_POINT('Ctrl Pts',(3.6681299835651,-42.6742356128,1.77956437899082));
#72470=CARTESIAN_POINT('Ctrl Pts',(3.82433912948244,-42.6742356128,1.86588929707841));
#72471=CARTESIAN_POINT('Ctrl Pts',(3.98280673611594,-42.6742356128,1.95346229468901));
#72472=CARTESIAN_POINT('Ctrl Pts',(4.14511704822198,-42.6742356128,2.03410582589879));
#72473=CARTESIAN_POINT('Ctrl Pts',(4.31063811976049,-42.6742356128,2.1074981892179));
#72474=CARTESIAN_POINT('Ctrl Pts',(4.47978318815511,-42.6742356128,2.18249743975359));
#72475=CARTESIAN_POINT('Ctrl Pts',(4.65228095758631,-42.6742356128,2.24992450648734));
#72476=CARTESIAN_POINT('Ctrl Pts',(4.82742445854302,-42.6742356128,2.30947944587345));
#72477=CARTESIAN_POINT('Ctrl Pts',(4.86342784939903,-42.6742356128,2.32172186279678));
#72478=CARTESIAN_POINT('Ctrl Pts',(4.8995429390839,-42.6742356128,2.33363177089508));
#72479=CARTESIAN_POINT('Ctrl Pts',(4.9357634328988,-42.6742356128,2.34520678581771));
#72480=CARTESIAN_POINT('Ctrl Pts',(4.9509736781236,-42.6742356128,2.35006753720209));
#72481=CARTESIAN_POINT('Ctrl Pts',(4.96620142604667,-42.6742356128,2.35486889455));
#72482=CARTESIAN_POINT('Ctrl Pts',(4.98144914733,-42.6742356128,2.3596116021));
#72483=CARTESIAN_POINT('',(-0.779760475483967,-42.6742356128,-2.17482015902982));
#72484=CARTESIAN_POINT('Ctrl Pts',(-0.779760436124172,-42.6742356128,-2.1748203306699));
#72485=CARTESIAN_POINT('Ctrl Pts',(-0.771882386024557,-42.6742356128,-2.2091747844539));
#72486=CARTESIAN_POINT('Ctrl Pts',(-0.761743310786152,-42.6742356127436,
-2.24303459797053));
#72487=CARTESIAN_POINT('Ctrl Pts',(-0.749417245972666,-42.6742356121532,
-2.27609427848163));
#72488=CARTESIAN_POINT('Ctrl Pts',(-0.743947277564191,-42.6742356118913,
-2.29076525504441));
#72489=CARTESIAN_POINT('Ctrl Pts',(-0.738047224848478,-42.6742356115623,
-2.30527902661246));
#72490=CARTESIAN_POINT('Ctrl Pts',(-0.731726287300169,-42.6742356113417,
-2.31961063905224));
#72491=CARTESIAN_POINT('Ctrl Pts',(-0.71748704598615,-42.6742356108449,
-2.35189561044918));
#72492=CARTESIAN_POINT('Ctrl Pts',(-0.701108863892468,-42.6742356109896,
-2.38325168854725));
#72493=CARTESIAN_POINT('Ctrl Pts',(-0.682724258933874,-42.6742356115095,
-2.41339155273195));
#72494=CARTESIAN_POINT('Ctrl Pts',(-0.674556959324613,-42.6742356117405,
-2.42678108715671));
#72495=CARTESIAN_POINT('Ctrl Pts',(-0.665994299629919,-42.6742356120229,
-2.43993092853152));
#72496=CARTESIAN_POINT('Ctrl Pts',(-0.657050718113802,-42.6742356122661,
-2.45281754922215));
#72497=CARTESIAN_POINT('Ctrl Pts',(-0.636448244523914,-42.6742356128262,
-2.48250322514104));
#72498=CARTESIAN_POINT('Ctrl Pts',(-0.613815845819897,-42.6742356127802,
-2.5107827227237));
#72499=CARTESIAN_POINT('Ctrl Pts',(-0.589368331375716,-42.6742356127938,
-2.53739155422732));
#72500=CARTESIAN_POINT('Ctrl Pts',(-0.567203612838432,-42.6742356128062,
-2.56151577602625));
#72501=CARTESIAN_POINT('Ctrl Pts',(-0.543547753181066,-42.6742356128,-2.58426707716386));
#72502=CARTESIAN_POINT('Ctrl Pts',(-0.518587085338794,-42.6742356128,-2.60547441341678));
#72503=CARTESIAN_POINT('Ctrl Pts',(-0.4900008751542,-42.6742356128,-2.62976211979596));
#72504=CARTESIAN_POINT('Ctrl Pts',(-0.459703825368212,-42.6742356128016,
-2.6520234184038));
#72505=CARTESIAN_POINT('Ctrl Pts',(-0.428000961425894,-42.6742356127984,
-2.67204333218478));
#72506=CARTESIAN_POINT('Ctrl Pts',(-0.396135658604291,-42.6742356127953,
-2.69216582383898));
#72507=CARTESIAN_POINT('Ctrl Pts',(-0.362850627609383,-42.6742356128003,
-2.71002365359072));
#72508=CARTESIAN_POINT('Ctrl Pts',(-0.328481739610751,-42.6742356126976,
-2.72544414029683));
#72509=CARTESIAN_POINT('Ctrl Pts',(-0.302412698880465,-42.6742356126197,
-2.73714068677917));
#72510=CARTESIAN_POINT('Ctrl Pts',(-0.275720672999424,-42.674235612482,
-2.74743585589414));
#72511=CARTESIAN_POINT('Ctrl Pts',(-0.248559329784468,-42.6742356120918,
-2.75627299220266));
#72512=CARTESIAN_POINT('Ctrl Pts',(-0.213345963022923,-42.6742356115859,
-2.76772991167425));
#72513=CARTESIAN_POINT('Ctrl Pts',(-0.177343992087915,-42.6742356115549,
-2.77674513901392));
#72514=CARTESIAN_POINT('Ctrl Pts',(-0.140897295835687,-42.6742356118431,
-2.7832338109811));
#72515=CARTESIAN_POINT('Ctrl Pts',(-0.105167926379445,-42.6742356121256,
-2.78959477594734));
#72516=CARTESIAN_POINT('Ctrl Pts',(-0.0690116959894625,-42.6742356125303,
-2.79352757273382));
#72517=CARTESIAN_POINT('Ctrl Pts',(-0.0327575959623081,-42.6742356126816,
-2.79500142010586));
#72518=CARTESIAN_POINT('Ctrl Pts',(-0.00125856507985131,-42.674235612813,
-2.79628195841334));
#72519=CARTESIAN_POINT('Ctrl Pts',(0.0303140671195736,-42.6742356128,-2.79570693363651));
#72520=CARTESIAN_POINT('Ctrl Pts',(0.0617459707272592,-42.6742356128,-2.7932881369414));
#72521=CARTESIAN_POINT('Ctrl Pts',(0.0975001652207659,-42.6742356128,-2.79053672460072));
#72522=CARTESIAN_POINT('Ctrl Pts',(0.133074926050902,-42.6742356128188,
-2.78539779724224));
#72523=CARTESIAN_POINT('Ctrl Pts',(0.168152094213755,-42.6742356125744,
-2.77790104853703));
#72524=CARTESIAN_POINT('Ctrl Pts',(0.203937242420985,-42.674235612325,-2.77025298919988));
#72525=CARTESIAN_POINT('Ctrl Pts',(0.239204002026126,-42.6742356117404,
-2.76015111489368));
#72526=CARTESIAN_POINT('Ctrl Pts',(0.273621672102003,-42.6742356113681,
-2.74768128575085));
#72527=CARTESIAN_POINT('Ctrl Pts',(0.303967810871832,-42.6742356110398,
-2.73668660875005));
#72528=CARTESIAN_POINT('Ctrl Pts',(0.333653760938991,-42.6742356110113,
-2.72385202374141));
#72529=CARTESIAN_POINT('Ctrl Pts',(0.362462032603895,-42.6742356115161,
-2.70926867569233));
#72530=CARTESIAN_POINT('Ctrl Pts',(0.395399194544457,-42.6742356120931,
-2.69259519725825));
#72531=CARTESIAN_POINT('Ctrl Pts',(0.427186062002718,-42.6742356125277,
-2.67362882788146));
#72532=CARTESIAN_POINT('Ctrl Pts',(0.457510957670161,-42.6742356126845,
-2.65254442199209));
#72533=CARTESIAN_POINT('Ctrl Pts',(0.483644635797922,-42.6742356128196,
-2.63437410137267));
#72534=CARTESIAN_POINT('Ctrl Pts',(0.508692612723636,-42.6742356128,-2.61463163103994));
#72535=CARTESIAN_POINT('Ctrl Pts',(0.532470455680955,-42.6742356128,-2.59345610321658));
#72536=CARTESIAN_POINT('Ctrl Pts',(0.559653617309548,-42.6742356128,-2.56924794453598));
#72537=CARTESIAN_POINT('Ctrl Pts',(0.585178113150637,-42.674235612815,-2.54316956742759));
#72538=CARTESIAN_POINT('Ctrl Pts',(0.608798795510751,-42.6742356127792,
-2.51546647952722));
#72539=CARTESIAN_POINT('Ctrl Pts',(0.618869569523831,-42.6742356127639,
-2.50365515530484));
#72540=CARTESIAN_POINT('Ctrl Pts',(0.628594706907684,-42.6742356127371,
-2.4915489628781));
#72541=CARTESIAN_POINT('Ctrl Pts',(0.637957296244174,-42.6742356126657,
-2.47916894035594));
#72542=CARTESIAN_POINT('Ctrl Pts',(0.65952394751115,-42.6742356125014,-2.45065165535956));
#72543=CARTESIAN_POINT('Ctrl Pts',(0.679165969277145,-42.6742356121484,
-2.42068246401955));
#72544=CARTESIAN_POINT('Ctrl Pts',(0.696711688177922,-42.6742356119776,
-2.38954124508249));
#72545=CARTESIAN_POINT('Ctrl Pts',(0.704648211534099,-42.6742356119004,
-2.37545501625189));
#72546=CARTESIAN_POINT('Ctrl Pts',(0.712156407805598,-42.6742356118675,
-2.36112935270655));
#72547=CARTESIAN_POINT('Ctrl Pts',(0.719223465086762,-42.6742356119079,
-2.34659188406283));
#72548=CARTESIAN_POINT('Ctrl Pts',(0.734743304322684,-42.6742356119965,
-2.31466640684203));
#72549=CARTESIAN_POINT('Ctrl Pts',(0.748133092456025,-42.6742356124825,
-2.28172010730082));
#72550=CARTESIAN_POINT('Ctrl Pts',(0.759286157002397,-42.6742356126654,
-2.24805003279359));
#72551=CARTESIAN_POINT('Ctrl Pts',(0.764654983546271,-42.6742356127534,
-2.23184204000406));
#72552=CARTESIAN_POINT('Ctrl Pts',(0.76950616314712,-42.6742356127875,-2.21546668989043));
#72553=CARTESIAN_POINT('Ctrl Pts',(0.773831693881399,-42.6742356127965,
-2.19895906143653));
#72554=CARTESIAN_POINT('Ctrl Pts',(0.775495494440411,-42.6742356127999,
-2.19260945877808));
#72555=CARTESIAN_POINT('Ctrl Pts',(0.777081584877396,-42.6742356128,-2.18623986325737));
#72556=CARTESIAN_POINT('Ctrl Pts',(0.77858938947441,-42.6742356128,-2.17985291185987));
#72557=CARTESIAN_POINT('Ctrl Pts',(0.778985012316415,-42.6742356128,-2.17817708206825));
#72558=CARTESIAN_POINT('Ctrl Pts',(0.779375249835899,-42.6742356128,-2.17650001824316));
#72559=CARTESIAN_POINT('Ctrl Pts',(0.77975997749,-42.6742356128,-2.17482231881));
#72560=CARTESIAN_POINT('',(-4.9814499490356,-42.6742356128,2.35961185030861));
#72561=CARTESIAN_POINT('Ctrl Pts',(-4.98144948349564,-42.6742356128,2.35961170550494));
#72562=CARTESIAN_POINT('Ctrl Pts',(-4.80919836505199,-42.6742356128,2.30603390147258));
#72563=CARTESIAN_POINT('Ctrl Pts',(-4.63925280032748,-42.6742356128,2.24489003529727));
#72564=CARTESIAN_POINT('Ctrl Pts',(-4.47229043758232,-42.6742356128,2.17645227217075));
#72565=CARTESIAN_POINT('Ctrl Pts',(-4.30666840647509,-42.6742356128,2.10856391010469));
#72566=CARTESIAN_POINT('Ctrl Pts',(-4.1439818210772,-42.6742356128,2.03349814638391));
#72567=CARTESIAN_POINT('Ctrl Pts',(-3.9848542066517,-42.6742356128,1.95155469208076));
#72568=CARTESIAN_POINT('Ctrl Pts',(-3.82699882905798,-42.6742356128,1.87026638164477));
#72569=CARTESIAN_POINT('Ctrl Pts',(-3.67264569158656,-42.6742356128,1.78220978388477));
#72570=CARTESIAN_POINT('Ctrl Pts',(-3.52236675719064,-42.6742356128,1.68771315474634));
#72571=CARTESIAN_POINT('Ctrl Pts',(-3.37392108171852,-42.6742356128,1.59436929388734));
#72572=CARTESIAN_POINT('Ctrl Pts',(-3.22945074026306,-42.6742356128,1.49474147234454));
#72573=CARTESIAN_POINT('Ctrl Pts',(-3.08947198433951,-42.6742356128,1.38918267495346));
#72574=CARTESIAN_POINT('Ctrl Pts',(-2.95042677891965,-42.6742356128,1.28432787344963));
#72575=CARTESIAN_POINT('Ctrl Pts',(-2.81581340943447,-42.6742356128,1.17362082121951));
#72576=CARTESIAN_POINT('Ctrl Pts',(-2.68610386179253,-42.6742356128,1.05744547667766));
#72577=CARTESIAN_POINT('Ctrl Pts',(-2.55777390003295,-42.6742356128,0.942505768741767));
#72578=CARTESIAN_POINT('Ctrl Pts',(-2.43424394217692,-42.6742356128,0.822213384451512));
#72579=CARTESIAN_POINT('Ctrl Pts',(-2.31593843360122,-42.6742356128,0.696978970869958));
#72580=CARTESIAN_POINT('Ctrl Pts',(-2.21042894038762,-42.6742356128,0.585290008378093));
#72581=CARTESIAN_POINT('Ctrl Pts',(-2.10907441450449,-42.6742356128,0.469670718927621));
#72582=CARTESIAN_POINT('Ctrl Pts',(-2.01215415618858,-42.6742356128,0.35043979706303));
#72583=CARTESIAN_POINT('Ctrl Pts',(-1.9037090267106,-42.6742356128,0.217031023870963));
#72584=CARTESIAN_POINT('Ctrl Pts',(-1.80081569189617,-42.6742356128,0.0790993529284168));
#72585=CARTESIAN_POINT('Ctrl Pts',(-1.70382506592654,-42.6742356128,-0.062882265463112));
#72586=CARTESIAN_POINT('Ctrl Pts',(-1.60543636915258,-42.6742356128,-0.206910477053096));
#72587=CARTESIAN_POINT('Ctrl Pts',(-1.51312175751413,-42.6742356128,-0.355106089171734));
#72588=CARTESIAN_POINT('Ctrl Pts',(-1.42720569724974,-42.6742356128,-0.506941748698572));
#72589=CARTESIAN_POINT('Ctrl Pts',(-1.33928851382052,-42.6742356128,-0.662313904831416));
#72590=CARTESIAN_POINT('Ctrl Pts',(-1.25807145212962,-42.6742356128,-0.821497524831694));
#72591=CARTESIAN_POINT('Ctrl Pts',(-1.18385847761663,-42.6742356128,-0.983894534460413));
#72592=CARTESIAN_POINT('Ctrl Pts',(-1.10857063815684,-42.6742356128,-1.14864362408946));
#72593=CARTESIAN_POINT('Ctrl Pts',(-1.04049120426499,-42.6742356128,-1.31669966268174));
#72594=CARTESIAN_POINT('Ctrl Pts',(-0.979893200082159,-42.6742356128,-1.48740715124177));
#72595=CARTESIAN_POINT('Ctrl Pts',(-0.939948615418486,-42.6742356128,-1.59993296494573));
#72596=CARTESIAN_POINT('Ctrl Pts',(-0.903253871668043,-42.6742356128,-1.71361022529542));
#72597=CARTESIAN_POINT('Ctrl Pts',(-0.869877025508678,-42.6742356128,-1.82824463543011));
#72598=CARTESIAN_POINT('Ctrl Pts',(-0.85185246901731,-42.6742356128,-1.8901508560317));
#72599=CARTESIAN_POINT('Ctrl Pts',(-0.834795388868271,-42.6742356128,-1.95233612918722));
#72600=CARTESIAN_POINT('Ctrl Pts',(-0.81871556018869,-42.6742356128,-2.01476928736231));
#72601=CARTESIAN_POINT('Ctrl Pts',(-0.807621905288932,-42.6742356128,-2.05784262631996));
#72602=CARTESIAN_POINT('Ctrl Pts',(-0.796993187080195,-42.6742356128,-2.10103480337359));
#72603=CARTESIAN_POINT('Ctrl Pts',(-0.786833098471183,-42.6742356128,-2.14433263155088));
#72604=CARTESIAN_POINT('Ctrl Pts',(-0.784449857609889,-42.6742356128,-2.15448895570202));
#72605=CARTESIAN_POINT('Ctrl Pts',(-0.78209237975105,-42.6742356128,-2.16465117321392));
#72606=CARTESIAN_POINT('Ctrl Pts',(-0.779760514736,-42.6742356128,-2.17481998786));
#72607=CARTESIAN_POINT('',(-5.54384247076,-42.6742356128,3.12351150632));
#72608=CARTESIAN_POINT('Ctrl Pts',(-5.54384247076,-42.6742356128,3.12351150632));
#72609=CARTESIAN_POINT('Ctrl Pts',(-5.54384247076,-42.6742356128,3.08277773492765));
#72610=CARTESIAN_POINT('Ctrl Pts',(-5.54071360078215,-42.6742356128,3.04207318197935));
#72611=CARTESIAN_POINT('Ctrl Pts',(-5.53451433673871,-42.6742356128,3.00184928981549));
#72612=CARTESIAN_POINT('Ctrl Pts',(-5.52845684412169,-42.6742356128,2.96254528080684));
#72613=CARTESIAN_POINT('Ctrl Pts',(-5.51946761052196,-42.6742356128,2.92370108139371));
#72614=CARTESIAN_POINT('Ctrl Pts',(-5.50764984198096,-42.6742356128,2.88573839093141));
#72615=CARTESIAN_POINT('Ctrl Pts',(-5.49633599201714,-42.6742356128,2.84939445826564));
#72616=CARTESIAN_POINT('Ctrl Pts',(-5.48242970534344,-42.6742356128,2.81385906698573));
#72617=CARTESIAN_POINT('Ctrl Pts',(-5.46606736204047,-42.6742356128,2.77949183965844));
#72618=CARTESIAN_POINT('Ctrl Pts',(-5.45540608526423,-42.6742356128,2.75709904934816));
#72619=CARTESIAN_POINT('Ctrl Pts',(-5.44370303413002,-42.6742356128,2.73520201301567));
#72620=CARTESIAN_POINT('Ctrl Pts',(-5.43100715596564,-42.6742356128,2.71389584592905));
#72621=CARTESIAN_POINT('Ctrl Pts',(-5.41253132965188,-42.6742356128,2.68288979519291));
#72622=CARTESIAN_POINT('Ctrl Pts',(-5.39195153436773,-42.6742356128,2.65313745264134));
#72623=CARTESIAN_POINT('Ctrl Pts',(-5.36945481472739,-42.6742356128,2.62491223520097));
#72624=CARTESIAN_POINT('Ctrl Pts',(-5.36214844037038,-42.6742356128,2.61574538740164));
#72625=CARTESIAN_POINT('Ctrl Pts',(-5.3546402157141,-42.6742356128,2.60673941007348));
#72626=CARTESIAN_POINT('Ctrl Pts',(-5.34693756224094,-42.6742356128,2.59790301992746));
#72627=CARTESIAN_POINT('Ctrl Pts',(-5.32245762826908,-42.6742356128,2.56981993815857));
#72628=CARTESIAN_POINT('Ctrl Pts',(-5.29601080618723,-42.6742356128,2.54345222915515));
#72629=CARTESIAN_POINT('Ctrl Pts',(-5.26786034544883,-42.6742356127988,
2.519055298754));
#72630=CARTESIAN_POINT('Ctrl Pts',(-5.23866597118581,-42.6742356127975,
2.49375364832564));
#72631=CARTESIAN_POINT('Ctrl Pts',(-5.20763878578798,-42.674235612795,2.47057122522464));
#72632=CARTESIAN_POINT('Ctrl Pts',(-5.17509880313699,-42.6742356127955,
2.44974305729505));
#72633=CARTESIAN_POINT('Ctrl Pts',(-5.15847322776628,-42.6742356127958,
2.43910137135866));
#72634=CARTESIAN_POINT('Ctrl Pts',(-5.14145320351809,-42.674235612797,2.42907350989681));
#72635=CARTESIAN_POINT('Ctrl Pts',(-5.1240845467918,-42.6742356127983,2.41968668236892));
#72636=CARTESIAN_POINT('Ctrl Pts',(-5.08693883187455,-42.6742356128011,
2.39961141547735));
#72637=CARTESIAN_POINT('Ctrl Pts',(-5.04819985954546,-42.6742356128,2.38247336856776));
#72638=CARTESIAN_POINT('Ctrl Pts',(-5.00832557034011,-42.6742356128,2.36849837699853));
#72639=CARTESIAN_POINT('Ctrl Pts',(-5.00019121922974,-42.6742356128,2.36564748008089));
#72640=CARTESIAN_POINT('Ctrl Pts',(-4.99200978031334,-42.6742356128,2.36292815045189));
#72641=CARTESIAN_POINT('Ctrl Pts',(-4.98378540040244,-42.6742356128,2.36034222294903));
#72642=CARTESIAN_POINT('Ctrl Pts',(-4.98300737166342,-42.6742356128,2.36009759345282));
#72643=CARTESIAN_POINT('Ctrl Pts',(-4.98222894973333,-42.6742356128,2.35985415528));
#72644=CARTESIAN_POINT('Ctrl Pts',(-4.98145041415,-42.6742356128,2.35961199498));
#72645=CARTESIAN_POINT('',(-5.54384247374,-42.6742356128,6.92092019865));
#72646=CARTESIAN_POINT('',(-5.54384247076,-42.6742356128,1.77756718468));
#72647=CARTESIAN_POINT('',(1.46955156614709E-7,-42.6742356128,12.4643460018));
#72648=CARTESIAN_POINT('Ctrl Pts',(2.6645352591E-15,-42.6742356128,12.4643460018));
#72649=CARTESIAN_POINT('Ctrl Pts',(-0.152934422951822,-42.6742356128,12.4643459942906));
#72650=CARTESIAN_POINT('Ctrl Pts',(-0.305879899778285,-42.6742356128,12.4580345127897));
#72651=CARTESIAN_POINT('Ctrl Pts',(-0.458305068588312,-42.6742356128,12.4454167663129));
#72652=CARTESIAN_POINT('Ctrl Pts',(-0.612162616952914,-42.6742356128,12.4326804475411));
#72653=CARTESIAN_POINT('Ctrl Pts',(-0.765489828123542,-42.6742356128,12.4135188817167));
#72654=CARTESIAN_POINT('Ctrl Pts',(-0.917747353463392,-42.6742356128,12.3879900366151));
#72655=CARTESIAN_POINT('Ctrl Pts',(-1.07200490475462,-42.6742356128,12.3621258494502));
#72656=CARTESIAN_POINT('Ctrl Pts',(-1.22516425528739,-42.6742356128,12.3297260830963));
#72657=CARTESIAN_POINT('Ctrl Pts',(-1.37667510471216,-42.6742356128,12.2909034822149));
#72658=CARTESIAN_POINT('Ctrl Pts',(-1.52925372735887,-42.6742356128,12.2518072789229));
#72659=CARTESIAN_POINT('Ctrl Pts',(-1.68016030056891,-42.6742356128,12.2061975321192));
#72660=CARTESIAN_POINT('Ctrl Pts',(-1.82884693378749,-42.6742356128,12.15424051866));
#72661=CARTESIAN_POINT('Ctrl Pts',(-1.97886109712591,-42.6742356128,12.1018196134655));
#72662=CARTESIAN_POINT('Ctrl Pts',(-2.12661525264074,-42.6742356128,12.0429377287266));
#72663=CARTESIAN_POINT('Ctrl Pts',(-2.27156468105575,-42.6742356128,11.9778154451136));
#72664=CARTESIAN_POINT('Ctrl Pts',(-2.30699184911197,-42.6742356128,11.9618988726166));
#72665=CARTESIAN_POINT('Ctrl Pts',(-2.34225156607063,-42.6742356128,11.9456097462612));
#72666=CARTESIAN_POINT('Ctrl Pts',(-2.37733606672488,-42.6742356128,11.9289517189297));
#72667=CARTESIAN_POINT('Ctrl Pts',(-2.52218856563558,-42.6742356128,11.8601761388049));
#72668=CARTESIAN_POINT('Ctrl Pts',(-2.66405185080705,-42.6742356128,11.7851089263726));
#72669=CARTESIAN_POINT('Ctrl Pts',(-2.8023946521394,-42.6742356128,11.7040363137361));
#72670=CARTESIAN_POINT('Ctrl Pts',(-2.94501320772194,-42.6742356128,11.6204579937933));
#72671=CARTESIAN_POINT('Ctrl Pts',(-3.08388989194594,-42.6742356128,11.5304973181011));
#72672=CARTESIAN_POINT('Ctrl Pts',(-3.21847226185907,-42.6742356128,11.4345172231166));
#72673=CARTESIAN_POINT('Ctrl Pts',(-3.3499760674468,-42.6742356128,11.3407326675371));
#72674=CARTESIAN_POINT('Ctrl Pts',(-3.47737964611668,-42.6742356128,11.2412013333675));
#72675=CARTESIAN_POINT('Ctrl Pts',(-3.60019907306528,-42.6742356128,11.1363045235771));
#72676=CARTESIAN_POINT('Ctrl Pts',(-3.7273313885791,-42.6742356128,11.0277241902375));
#72677=CARTESIAN_POINT('Ctrl Pts',(-3.84955145038418,-42.6742356128,10.9133949502508));
#72678=CARTESIAN_POINT('Ctrl Pts',(-3.96636185003895,-42.6742356128,10.7937834186627));
#72679=CARTESIAN_POINT('Ctrl Pts',(-4.08317224969372,-42.6742356128,10.6741718870745));
#72680=CARTESIAN_POINT('Ctrl Pts',(-4.19457269676896,-42.6742356128,10.5492783343306));
#72681=CARTESIAN_POINT('Ctrl Pts',(-4.30011007911526,-42.6742356128,10.4196098288233));
#72682=CARTESIAN_POINT('Ctrl Pts',(-4.40180740998025,-42.6742356128,10.2946594025935));
#72683=CARTESIAN_POINT('Ctrl Pts',(-4.49805952609308,-42.6742356128,10.1652770827442));
#72684=CARTESIAN_POINT('Ctrl Pts',(-4.58849736625876,-42.6742356128,10.031953943456));
#72685=CARTESIAN_POINT('Ctrl Pts',(-4.67853934273498,-42.6742356128,9.89921438499756));
#72686=CARTESIAN_POINT('Ctrl Pts',(-4.76281768342982,-42.6742356128,9.76256862347885));
#72687=CARTESIAN_POINT('Ctrl Pts',(-4.84101173146805,-42.6742356128,9.62252848262185));
#72688=CARTESIAN_POINT('Ctrl Pts',(-4.9188015286105,-42.6742356128,9.48321232720629));
#72689=CARTESIAN_POINT('Ctrl Pts',(-4.9905696427724,-42.6742356128,9.34053698753787));
#72690=CARTESIAN_POINT('Ctrl Pts',(-5.05604571341481,-42.6742356128,9.19503049048107));
#72691=CARTESIAN_POINT('Ctrl Pts',(-5.12113898989817,-42.6742356128,9.05037467118533));
#72692=CARTESIAN_POINT('Ctrl Pts',(-5.18001345232591,-42.6742356128,8.90292088539472));
#72693=CARTESIAN_POINT('Ctrl Pts',(-5.23245034475332,-42.6742356128,8.75320905292079));
#72694=CARTESIAN_POINT('Ctrl Pts',(-5.28435356154415,-42.6742356128,8.60502091023473));
#72695=CARTESIAN_POINT('Ctrl Pts',(-5.32994949468892,-42.6742356128,8.4546206362449));
#72696=CARTESIAN_POINT('Ctrl Pts',(-5.3690735764806,-42.6742356128,8.30254979313354));
#72697=CARTESIAN_POINT('Ctrl Pts',(-5.4079616738089,-42.6742356128,8.15139619471301));
#72698=CARTESIAN_POINT('Ctrl Pts',(-5.440455646721,-42.6742356128,7.99859228485633));
#72699=CARTESIAN_POINT('Ctrl Pts',(-5.46644261980943,-42.6742356128,7.8446851206844));
#72700=CARTESIAN_POINT('Ctrl Pts',(-5.49215843779819,-42.6742356128,7.69238386545387));
#72701=CARTESIAN_POINT('Ctrl Pts',(-5.5115022728444,-42.6742356128,7.53900242459925));
#72702=CARTESIAN_POINT('Ctrl Pts',(-5.52441386329599,-42.6742356128,7.3850834002636));
#72703=CARTESIAN_POINT('Ctrl Pts',(-5.53701510708161,-42.6742356128,7.23486401744098));
#72704=CARTESIAN_POINT('Ctrl Pts',(-5.54348965896334,-42.6742356128,7.0841327522232));
#72705=CARTESIAN_POINT('Ctrl Pts',(-5.54382843698574,-42.6742356128,6.93340348714827));
#72706=CARTESIAN_POINT('Ctrl Pts',(-5.54383778962934,-42.6742356128,6.92924230489017));
#72707=CARTESIAN_POINT('Ctrl Pts',(-5.54384246875505,-42.6742356128,6.92508112888333));
#72708=CARTESIAN_POINT('Ctrl Pts',(-5.54384247523,-42.6742356128,6.92092019865));
#72709=CARTESIAN_POINT('Ctrl Pts',(5.54384244762,-42.6742356128,6.92091963994));
#72710=CARTESIAN_POINT('Ctrl Pts',(5.54384243194334,-42.6742356128,6.92966373948699));
#72711=CARTESIAN_POINT('Ctrl Pts',(5.54382181063784,-42.6742356128,6.93840868167453));
#72712=CARTESIAN_POINT('Ctrl Pts',(5.5437805349069,-42.6742356128,6.94715314260851));
#72713=CARTESIAN_POINT('Ctrl Pts',(5.54305520621443,-42.6742356128,7.10081749384282));
#72714=CARTESIAN_POINT('Ctrl Pts',(5.53595215261845,-42.6742356128,7.25446554541178));
#72715=CARTESIAN_POINT('Ctrl Pts',(5.52248273569997,-42.6742356128,7.40755466122751));
#72716=CARTESIAN_POINT('Ctrl Pts',(5.50836100597807,-42.6742356128,7.56805775724128));
#72717=CARTESIAN_POINT('Ctrl Pts',(5.48724107786514,-42.6742356128,7.72794619824574));
#72718=CARTESIAN_POINT('Ctrl Pts',(5.45919555961385,-42.6742356128,7.88660567787795));
#72719=CARTESIAN_POINT('Ctrl Pts',(5.43185920864886,-42.6742356128,8.04125324688654));
#72720=CARTESIAN_POINT('Ctrl Pts',(5.39794349973922,-42.6742356128,8.19473309461251));
#72721=CARTESIAN_POINT('Ctrl Pts',(5.35756863797163,-42.6742356128,8.34648936004158));
#72722=CARTESIAN_POINT('Ctrl Pts',(5.31689946083409,-42.6742356128,8.49935186334855));
#72723=CARTESIAN_POINT('Ctrl Pts',(5.26967674106624,-42.6742356128,8.65046536546907));
#72724=CARTESIAN_POINT('Ctrl Pts',(5.21607418264677,-42.6742356128,8.79927766128295));
#72725=CARTESIAN_POINT('Ctrl Pts',(5.16211508332785,-42.6742356128,8.94907979174951));
#72726=CARTESIAN_POINT('Ctrl Pts',(5.10169112673359,-42.6742356128,9.0965497937351));
#72727=CARTESIAN_POINT('Ctrl Pts',(5.03502889143353,-42.6742356128,9.24114349268404));
#72728=CARTESIAN_POINT('Ctrl Pts',(4.9666514619051,-42.6742356128,9.3894575330944));
#72729=CARTESIAN_POINT('Ctrl Pts',(4.89171060292642,-42.6742356128,9.53474504778954));
#72730=CARTESIAN_POINT('Ctrl Pts',(4.81050183666432,-42.6742356128,9.67644283944644));
#72731=CARTESIAN_POINT('Ctrl Pts',(4.7303262629303,-42.6742356128,9.8163378565222));
#72732=CARTESIAN_POINT('Ctrl Pts',(4.64404156366582,-42.6742356128,9.9527337636317));
#72733=CARTESIAN_POINT('Ctrl Pts',(4.55197842717089,-42.6742356128,10.0851149237367));
#72734=CARTESIAN_POINT('Ctrl Pts',(4.45813571604418,-42.6742356128,10.2200550033312));
#72735=CARTESIAN_POINT('Ctrl Pts',(4.35828908770674,-42.6742356128,10.3508233132124));
#72736=CARTESIAN_POINT('Ctrl Pts',(4.25283467714301,-42.6742356128,10.4769049601158));
#72737=CARTESIAN_POINT('Ctrl Pts',(4.14738026657929,-42.6742356128,10.6029866070193));
#72738=CARTESIAN_POINT('Ctrl Pts',(4.03631829777995,-42.6742356128,10.7243813702904));
#72739=CARTESIAN_POINT('Ctrl Pts',(3.92008790027254,-42.6742356128,10.8406091727226));
#72740=CARTESIAN_POINT('Ctrl Pts',(3.80548814794816,-42.6742356128,10.9552063663791));
#72741=CARTESIAN_POINT('Ctrl Pts',(3.68586534857264,-42.6742356128,11.0647793545833));
#72742=CARTESIAN_POINT('Ctrl Pts',(3.56167933530323,-42.6742356128,11.1689068773146));
#72743=CARTESIAN_POINT('Ctrl Pts',(3.4379919014801,-42.6742356128,11.2726163510141));
#72744=CARTESIAN_POINT('Ctrl Pts',(3.309778046148,-42.6742356128,11.3709238168171));
#72745=CARTESIAN_POINT('Ctrl Pts',(3.17752456376651,-42.6742356128,11.4634531338962));
#72746=CARTESIAN_POINT('Ctrl Pts',(3.04581089145029,-42.6742356128,11.5556047803401));
#72747=CARTESIAN_POINT('Ctrl Pts',(2.91009072040676,-42.6742356128,11.6420251771074));
#72748=CARTESIAN_POINT('Ctrl Pts',(2.77087386987523,-42.6742356128,11.7223852197934));
#72749=CARTESIAN_POINT('Ctrl Pts',(2.63237555232269,-42.6742356128,11.8023305042037));
#72750=CARTESIAN_POINT('Ctrl Pts',(2.49041677304819,-42.6742356128,11.8762776720779));
#72751=CARTESIAN_POINT('Ctrl Pts',(2.34552496533561,-42.6742356128,11.9439472520736));
#72752=CARTESIAN_POINT('Ctrl Pts',(2.20151495801616,-42.6742356128,12.0112050002121));
#72753=CARTESIAN_POINT('Ctrl Pts',(2.05460772523369,-42.6742356128,12.0722611930782));
#72754=CARTESIAN_POINT('Ctrl Pts',(1.90534316243217,-42.6742356128,12.1268878184385));
#72755=CARTESIAN_POINT('Ctrl Pts',(1.75315419905355,-42.6742356128,12.1825846920327));
#72756=CARTESIAN_POINT('Ctrl Pts',(1.59851476541057,-42.6742356128,12.2315972208754));
#72757=CARTESIAN_POINT('Ctrl Pts',(1.4420176011676,-42.6742356128,12.273736305035));
#72758=CARTESIAN_POINT('Ctrl Pts',(1.29127071052453,-42.6742356128,12.3143270463583));
#72759=CARTESIAN_POINT('Ctrl Pts',(1.1388003798863,-42.6742356128,12.3485403027653));
#72760=CARTESIAN_POINT('Ctrl Pts',(0.985151863989862,-42.6742356128,12.3762563568521));
#72761=CARTESIAN_POINT('Ctrl Pts',(0.832564790435014,-42.6742356128,12.4037809415116));
#72762=CARTESIAN_POINT('Ctrl Pts',(0.678815934744325,-42.6742356128,12.4248976698191));
#72763=CARTESIAN_POINT('Ctrl Pts',(0.524451633473361,-42.6742356128,12.4395390775479));
#72764=CARTESIAN_POINT('Ctrl Pts',(0.43730184594899,-42.6742356128,12.4478052087849));
#72765=CARTESIAN_POINT('Ctrl Pts',(0.349956098267065,-42.6742356128,12.454008297127));
#72766=CARTESIAN_POINT('Ctrl Pts',(0.262514127733032,-42.6742356128,12.4581434972064));
#72767=CARTESIAN_POINT('Ctrl Pts',(0.212960826973561,-42.6742356128,12.4604869120676));
#72768=CARTESIAN_POINT('Ctrl Pts',(0.163376641704469,-42.6742356128,12.4621663256812));
#72769=CARTESIAN_POINT('Ctrl Pts',(0.113779847635199,-42.6742356128,12.4631816295884));
#72770=CARTESIAN_POINT('Ctrl Pts',(0.0806814244047195,-42.6742356128,12.4638591927063));
#72771=CARTESIAN_POINT('Ctrl Pts',(0.047577387565802,-42.6742356128,12.4642410020864));
#72772=CARTESIAN_POINT('Ctrl Pts',(0.0144731887327847,-42.6742356128,12.4643271664958));
#72773=CARTESIAN_POINT('Ctrl Pts',(0.0096488453239203,-42.6742356128,12.4643397234135));
#72774=CARTESIAN_POINT('Ctrl Pts',(0.00482444203328454,-42.6742356128,12.4643460015574));
#72775=CARTESIAN_POINT('Ctrl Pts',(2.93507693704953E-7,-42.6742356128,12.4643460018));
#72776=CARTESIAN_POINT('',(1.02290383517,-42.6742356128,-3.56061176027));
#72777=CARTESIAN_POINT('Origin',(6.82290383517,-42.6742356128,-3.56061176027));
#72778=CARTESIAN_POINT('',(-1.02290383517,-42.6742356128,-3.56061176027));
#72779=CARTESIAN_POINT('Origin',(-6.82290383517,-42.6742356128,-3.56061176027));
#72780=CARTESIAN_POINT('Origin',(-3.35265884719E-30,-40.6742356128,3.15283103411E-22));
#72781=CARTESIAN_POINT('',(6.74948971107,-40.6742356128,2.9389736393));
#72782=CARTESIAN_POINT('',(6.24384247076,-40.6742356128,3.43894174696));
#72783=CARTESIAN_POINT('Ctrl Pts',(6.74948971107,-40.6742356128,2.9389736393));
#72784=CARTESIAN_POINT('Ctrl Pts',(6.59129069763,-40.6742356128,2.93718674963));
#72785=CARTESIAN_POINT('Ctrl Pts',(6.43081292755,-40.6742356128,2.99918925876));
#72786=CARTESIAN_POINT('Ctrl Pts',(6.30765353814,-40.6742356128,3.12096539428));
#72787=CARTESIAN_POINT('Ctrl Pts',(6.24384247076,-40.6742356128,3.28073264221));
#72788=CARTESIAN_POINT('Ctrl Pts',(6.24384247076,-40.6742356128,3.43894174696));
#72789=CARTESIAN_POINT('',(0.4871654368,-40.6742356128,-5.0126513422));
#72790=CARTESIAN_POINT('Ctrl Pts',(0.4871654368,-40.6742356128,-5.0126513422));
#72791=CARTESIAN_POINT('Ctrl Pts',(0.813757598474,-40.6742356128,-6.43768308726));
#72792=CARTESIAN_POINT('Ctrl Pts',(1.54099672242,-40.6742356128,-7.77089360944));
#72793=CARTESIAN_POINT('Ctrl Pts',(2.63582398808,-40.6742356128,-8.86093046307));
#72794=CARTESIAN_POINT('Ctrl Pts',(5.30859738244,-40.6742356128,-10.303702289));
#72795=CARTESIAN_POINT('Ctrl Pts',(8.3416246802,-40.6742356128,-10.1422911046));
#72796=CARTESIAN_POINT('Ctrl Pts',(9.79740146658,-40.6742356128,-9.62504741726));
#72797=CARTESIAN_POINT('Ctrl Pts',(12.2523240225,-40.6742356128,-7.83656666427));
#72798=CARTESIAN_POINT('Ctrl Pts',(13.4155860878,-40.6742356128,-5.03083511496));
#72799=CARTESIAN_POINT('Ctrl Pts',(13.5772083053,-40.6742356128,-3.49437641304));
#72800=CARTESIAN_POINT('Ctrl Pts',(13.0232255151,-40.6742356128,-0.50800550047));
#72801=CARTESIAN_POINT('Ctrl Pts',(10.9941845663,-40.6742356128,1.75214958001));
#72802=CARTESIAN_POINT('Ctrl Pts',(9.67790042305,-40.6742356128,2.56099019349));
#72803=CARTESIAN_POINT('Ctrl Pts',(8.21137385808,-40.6742356128,2.95548591471));
#72804=CARTESIAN_POINT('Ctrl Pts',(6.74948971107,-40.6742356128,2.9389736393));
#72805=CARTESIAN_POINT('',(-6.66133814775E-16,-40.6742356128,-4.62434669465));
#72806=CARTESIAN_POINT('Ctrl Pts',(-6.66133814775E-16,-40.6742356128,-4.62434669465));
#72807=CARTESIAN_POINT('Ctrl Pts',(0.134351406801,-40.6742356128,-4.62434669465));
#72808=CARTESIAN_POINT('Ctrl Pts',(0.269654391195,-40.6742356128,-4.67008903963));
#72809=CARTESIAN_POINT('Ctrl Pts',(0.38229629568,-40.6742356128,-4.75983578098));
#72810=CARTESIAN_POINT('Ctrl Pts',(0.457108114206,-40.6742356128,-4.88150110685));
#72811=CARTESIAN_POINT('Ctrl Pts',(0.4871654368,-40.6742356128,-5.0126513422));
#72812=CARTESIAN_POINT('',(-0.4871654368,-40.6742356128,-5.0126513422));
#72813=CARTESIAN_POINT('Ctrl Pts',(-0.4871654368,-40.6742356128,-5.0126513422));
#72814=CARTESIAN_POINT('Ctrl Pts',(-0.457108114206,-40.6742356128,-4.88150110685));
#72815=CARTESIAN_POINT('Ctrl Pts',(-0.38229629568,-40.6742356128,-4.75983578098));
#72816=CARTESIAN_POINT('Ctrl Pts',(-0.269654391195,-40.6742356128,-4.67008903963));
#72817=CARTESIAN_POINT('Ctrl Pts',(-0.134351406801,-40.6742356128,-4.62434669465));
#72818=CARTESIAN_POINT('Ctrl Pts',(-6.66133814775E-16,-40.6742356128,-4.62434669465));
#72819=CARTESIAN_POINT('',(-6.74948971107,-40.6742356128,2.9389736393));
#72820=CARTESIAN_POINT('Ctrl Pts',(-6.74948971107,-40.6742356128,2.9389736393));
#72821=CARTESIAN_POINT('Ctrl Pts',(-8.21137385808,-40.6742356128,2.95548591471));
#72822=CARTESIAN_POINT('Ctrl Pts',(-9.67790042305,-40.6742356128,2.56099019349));
#72823=CARTESIAN_POINT('Ctrl Pts',(-10.9941845663,-40.6742356128,1.75214958001));
#72824=CARTESIAN_POINT('Ctrl Pts',(-13.0232255151,-40.6742356128,-0.50800550047));
#72825=CARTESIAN_POINT('Ctrl Pts',(-13.5772083053,-40.6742356128,-3.49437641304));
#72826=CARTESIAN_POINT('Ctrl Pts',(-13.4155860878,-40.6742356128,-5.03083511496));
#72827=CARTESIAN_POINT('Ctrl Pts',(-12.2523240225,-40.6742356128,-7.83656666427));
#72828=CARTESIAN_POINT('Ctrl Pts',(-9.79740146658,-40.6742356128,-9.62504741726));
#72829=CARTESIAN_POINT('Ctrl Pts',(-8.3416246802,-40.6742356128,-10.1422911046));
#72830=CARTESIAN_POINT('Ctrl Pts',(-5.30859738244,-40.6742356128,-10.303702289));
#72831=CARTESIAN_POINT('Ctrl Pts',(-2.63582398808,-40.6742356128,-8.86093046307));
#72832=CARTESIAN_POINT('Ctrl Pts',(-1.54099672242,-40.6742356128,-7.77089360944));
#72833=CARTESIAN_POINT('Ctrl Pts',(-0.813757598474,-40.6742356128,-6.43768308726));
#72834=CARTESIAN_POINT('Ctrl Pts',(-0.4871654368,-40.6742356128,-5.0126513422));
#72835=CARTESIAN_POINT('',(-6.24384247076,-40.6742356128,3.43894174696));
#72836=CARTESIAN_POINT('Ctrl Pts',(-6.24384247076,-40.6742356128,3.43894174696));
#72837=CARTESIAN_POINT('Ctrl Pts',(-6.24384247076,-40.6742356128,3.28073264221));
#72838=CARTESIAN_POINT('Ctrl Pts',(-6.30765353814,-40.6742356128,3.12096539428));
#72839=CARTESIAN_POINT('Ctrl Pts',(-6.43081292755,-40.6742356128,2.99918925876));
#72840=CARTESIAN_POINT('Ctrl Pts',(-6.59129069763,-40.6742356128,2.93718674963));
#72841=CARTESIAN_POINT('Ctrl Pts',(-6.74948971107,-40.6742356128,2.9389736393));
#72842=CARTESIAN_POINT('',(-6.24384247076,-40.6742356128,6.92091963994));
#72843=CARTESIAN_POINT('',(-6.24384247076,-40.6742356128,5.17993069345));
#72844=CARTESIAN_POINT('',(3.5527136788E-15,-40.6742356128,13.1643460036));
#72845=CARTESIAN_POINT('Ctrl Pts',(3.5527136788E-15,-40.6742356128,13.1643460036));
#72846=CARTESIAN_POINT('Ctrl Pts',(-1.96184634686,-40.6742356128,13.1643460036));
#72847=CARTESIAN_POINT('Ctrl Pts',(-3.92510661379,-40.6742356128,12.3963108842));
#72848=CARTESIAN_POINT('Ctrl Pts',(-5.47580735138,-40.6742356128,10.8456101466));
#72849=CARTESIAN_POINT('Ctrl Pts',(-6.24384247076,-40.6742356128,8.88234987966));
#72850=CARTESIAN_POINT('Ctrl Pts',(-6.24384247076,-40.6742356128,6.92091963994));
#72851=CARTESIAN_POINT('',(6.24384247076,-40.6742356128,6.92091963994));
#72852=CARTESIAN_POINT('Ctrl Pts',(6.24384247076,-40.6742356128,6.92091963994));
#72853=CARTESIAN_POINT('Ctrl Pts',(6.24384247076,-40.6742356128,8.88234987966));
#72854=CARTESIAN_POINT('Ctrl Pts',(5.47580735138,-40.6742356128,10.8456101466));
#72855=CARTESIAN_POINT('Ctrl Pts',(3.92510661379,-40.6742356128,12.3963108842));
#72856=CARTESIAN_POINT('Ctrl Pts',(1.96184634686,-40.6742356128,13.1643460036));
#72857=CARTESIAN_POINT('Ctrl Pts',(3.5527136788E-15,-40.6742356128,13.1643460036));
#72858=CARTESIAN_POINT('',(6.24384247076,-40.6742356128,5.17993069345));
#72859=CARTESIAN_POINT('',(-1.32290383517,-40.6742356128,-3.56061176027));
#72860=CARTESIAN_POINT('Origin',(-6.82290383517,-40.6742356128,-3.56061176027));
#72861=CARTESIAN_POINT('',(1.32290383517,-40.6742356128,-3.56061176027));
#72862=CARTESIAN_POINT('Origin',(6.82290383517,-40.6742356128,-3.56061176027));
#72863=CARTESIAN_POINT('',(4.89234685393,-40.6742356128,2.64607413014));
#72864=CARTESIAN_POINT('',(5.24384247076,-40.6742356128,3.12351150632));
#72865=CARTESIAN_POINT('Ctrl Pts',(4.89234685393,-40.6742356128,2.64607413014));
#72866=CARTESIAN_POINT('Ctrl Pts',(5.01354316676,-40.6742356128,2.6837716054));
#72867=CARTESIAN_POINT('Ctrl Pts',(5.12322496214,-40.6742356128,2.76042445737));
#72868=CARTESIAN_POINT('Ctrl Pts',(5.20322505246,-40.6742356128,2.86908878029));
#72869=CARTESIAN_POINT('Ctrl Pts',(5.24384247076,-40.6742356128,2.9965877265));
#72870=CARTESIAN_POINT('Ctrl Pts',(5.24384247076,-40.6742356128,3.12351150632));
#72871=CARTESIAN_POINT('',(5.24384247076,-40.6742356128,6.92091963994));
#72872=CARTESIAN_POINT('',(5.24384247076,-40.6742356128,5.02221557313));
#72873=CARTESIAN_POINT('',(3.10862446895E-15,-40.6742356128,12.1643460036));
#72874=CARTESIAN_POINT('Ctrl Pts',(5.24384247076,-40.6742356128,6.92091963994));
#72875=CARTESIAN_POINT('Ctrl Pts',(5.24384247076,-40.6742356128,8.5681906143));
#72876=CARTESIAN_POINT('Ctrl Pts',(4.59882235543,-40.6742356128,10.2169985032));
#72877=CARTESIAN_POINT('Ctrl Pts',(3.29649497043,-40.6742356128,11.5193258882));
#72878=CARTESIAN_POINT('Ctrl Pts',(1.64768708151,-40.6742356128,12.1643460036));
#72879=CARTESIAN_POINT('Ctrl Pts',(3.10862446895E-15,-40.6742356128,12.1643460036));
#72880=CARTESIAN_POINT('',(-5.24384247076,-40.6742356128,6.92091963994));
#72881=CARTESIAN_POINT('Ctrl Pts',(3.10862446895E-15,-40.6742356128,12.1643460036));
#72882=CARTESIAN_POINT('Ctrl Pts',(-1.64768708151,-40.6742356128,12.1643460036));
#72883=CARTESIAN_POINT('Ctrl Pts',(-3.29649497043,-40.6742356128,11.5193258882));
#72884=CARTESIAN_POINT('Ctrl Pts',(-4.59882235543,-40.6742356128,10.2169985032));
#72885=CARTESIAN_POINT('Ctrl Pts',(-5.24384247076,-40.6742356128,8.5681906143));
#72886=CARTESIAN_POINT('Ctrl Pts',(-5.24384247076,-40.6742356128,6.92091963994));
#72887=CARTESIAN_POINT('',(-5.24384247076,-40.6742356128,3.12351150632));
#72888=CARTESIAN_POINT('',(-5.24384247076,-40.6742356128,5.02221557313));
#72889=CARTESIAN_POINT('',(-4.89234685393,-40.6742356128,2.64607413014));
#72890=CARTESIAN_POINT('Ctrl Pts',(-5.24384247076,-40.6742356128,3.12351150632));
#72891=CARTESIAN_POINT('Ctrl Pts',(-5.24384247076,-40.6742356128,2.9965877265));
#72892=CARTESIAN_POINT('Ctrl Pts',(-5.20322505246,-40.6742356128,2.86908878029));
#72893=CARTESIAN_POINT('Ctrl Pts',(-5.12322496214,-40.6742356128,2.76042445737));
#72894=CARTESIAN_POINT('Ctrl Pts',(-5.01354316676,-40.6742356128,2.6837716054));
#72895=CARTESIAN_POINT('Ctrl Pts',(-4.89234685393,-40.6742356128,2.64607413014));
#72896=CARTESIAN_POINT('',(-0.48735027394,-40.6742356128,-2.10776590718));
#72897=CARTESIAN_POINT('Ctrl Pts',(-4.89234685393,-40.6742356128,2.64607413014));
#72898=CARTESIAN_POINT('Ctrl Pts',(-3.59661572838,-40.6742356128,2.2430437828));
#72899=CARTESIAN_POINT('Ctrl Pts',(-2.40362850687,-40.6742356128,1.49964984368));
#72900=CARTESIAN_POINT('Ctrl Pts',(-1.44114622406,-40.6742356128,0.46094601538));
#72901=CARTESIAN_POINT('Ctrl Pts',(-0.790651846747,-40.6742356128,-0.785131881257));
#72902=CARTESIAN_POINT('Ctrl Pts',(-0.48735027394,-40.6742356128,-2.10776590718));
#72903=CARTESIAN_POINT('',(0.48735027394,-40.6742356128,-2.10776590718));
#72904=CARTESIAN_POINT('Ctrl Pts',(-0.48735027394,-40.6742356128,-2.10776590718));
#72905=CARTESIAN_POINT('Ctrl Pts',(-0.427207937888,-40.6742356128,-2.37003391761));
#72906=CARTESIAN_POINT('Ctrl Pts',(-0.191539291907,-40.6742356128,-2.59726293898));
#72907=CARTESIAN_POINT('Ctrl Pts',(0.191539291907,-40.6742356128,-2.59726293898));
#72908=CARTESIAN_POINT('Ctrl Pts',(0.427207937888,-40.6742356128,-2.37003391761));
#72909=CARTESIAN_POINT('Ctrl Pts',(0.48735027394,-40.6742356128,-2.10776590718));
#72910=CARTESIAN_POINT('Ctrl Pts',(0.48735027394,-40.6742356128,-2.10776590718));
#72911=CARTESIAN_POINT('Ctrl Pts',(0.790651846747,-40.6742356128,-0.785131881257001));
#72912=CARTESIAN_POINT('Ctrl Pts',(1.44114622406,-40.6742356128,0.46094601538));
#72913=CARTESIAN_POINT('Ctrl Pts',(2.40362850687,-40.6742356128,1.49964984368));
#72914=CARTESIAN_POINT('Ctrl Pts',(3.59661572838,-40.6742356128,2.2430437828));
#72915=CARTESIAN_POINT('Ctrl Pts',(4.89234685393,-40.6742356128,2.64607413014));
#72916=CARTESIAN_POINT('Origin',(-6.82290383517,-42.3742356128,-3.56061176027));
#72917=CARTESIAN_POINT('',(-1.32290383517,-42.3742356128,-3.56061176027));
#72918=CARTESIAN_POINT('Origin',(-6.82290383517,-42.3742356128,-3.56061176027));
#72919=CARTESIAN_POINT('Origin',(-1.02290383517,-42.3742356128,-3.56061176027));
#72920=CARTESIAN_POINT('Origin',(-6.82290383517,-41.6742356128,-3.56061176027));
#72921=CARTESIAN_POINT('',(-1.32290383517,-41.6742356128,-3.56061176027));
#72922=CARTESIAN_POINT('Origin',(6.82290383517,-42.3742356128,-3.56061176027));
#72923=CARTESIAN_POINT('',(1.32290383517,-42.3742356128,-3.56061176027));
#72924=CARTESIAN_POINT('Origin',(6.82290383517,-42.3742356128,-3.56061176027));
#72925=CARTESIAN_POINT('Origin',(1.02290383517,-42.3742356128,-3.56061176027));
#72926=CARTESIAN_POINT('Origin',(6.82290383517,-41.6742356128,-3.56061176027));
#72927=CARTESIAN_POINT('',(1.32290383517,-41.6742356128,-3.56061176027));
#72928=CARTESIAN_POINT('Ctrl Pts',(4.98144948383,-42.6742356128,2.35961170443));
#72929=CARTESIAN_POINT('Ctrl Pts',(4.95345706708,-42.6742356128,2.44960652964));
#72930=CARTESIAN_POINT('Ctrl Pts',(4.92546465033,-42.6372245963,2.53960135485));
#72931=CARTESIAN_POINT('Ctrl Pts',(4.90333945028,-42.5627311721,2.61073324492));
#72932=CARTESIAN_POINT('Ctrl Pts',(4.89234685393,-42.4684833924,2.64607413014));
#72933=CARTESIAN_POINT('Ctrl Pts',(4.89234685393,-42.3742356128,2.64607413014));
#72934=CARTESIAN_POINT('Ctrl Pts',(5.0910703557,-42.6742356128,2.3937086997));
#72935=CARTESIAN_POINT('Ctrl Pts',(5.05009495057,-42.6742356128,2.4796652347));
#72936=CARTESIAN_POINT('Ctrl Pts',(5.00911954543,-42.6372245963,2.56562176971));
#72937=CARTESIAN_POINT('Ctrl Pts',(4.97673259252,-42.5627311721,2.63356179455));
#72938=CARTESIAN_POINT('Ctrl Pts',(4.96064159025,-42.4684833924,2.66731684844));
#72939=CARTESIAN_POINT('Ctrl Pts',(4.96064159025,-42.3742356128,2.66731684844));
#72940=CARTESIAN_POINT('Ctrl Pts',(5.19436346575,-42.6742356128,2.44749827577));
#72941=CARTESIAN_POINT('Ctrl Pts',(5.14132273239,-42.6742356128,2.52714226629));
#72942=CARTESIAN_POINT('Ctrl Pts',(5.08828199902,-42.6372245963,2.60678625681));
#72943=CARTESIAN_POINT('Ctrl Pts',(5.04635861923,-42.5627311721,2.6697368545));
#72944=CARTESIAN_POINT('Ctrl Pts',(5.02552956775,-42.4684833924,2.70101297135));
#72945=CARTESIAN_POINT('Ctrl Pts',(5.02552956775,-42.3742356128,2.70101297135));
#72946=CARTESIAN_POINT('Ctrl Pts',(5.28701136621,-42.6742356128,2.51927061523));
#72947=CARTESIAN_POINT('Ctrl Pts',(5.223039768,-42.6742356128,2.59047432619));
#72948=CARTESIAN_POINT('Ctrl Pts',(5.15906816979,-42.6372245963,2.66167803715));
#72949=CARTESIAN_POINT('Ctrl Pts',(5.10850502722,-42.5627311721,2.7179585308));
#72950=CARTESIAN_POINT('Ctrl Pts',(5.08338344476,-42.4684833924,2.74591906654));
#72951=CARTESIAN_POINT('Ctrl Pts',(5.08338344476,-42.3742356128,2.74591906654));
#72952=CARTESIAN_POINT('Ctrl Pts',(5.42454853942,-42.6742356128,2.67302418893));
#72953=CARTESIAN_POINT('Ctrl Pts',(5.34434320211,-42.6742356128,2.72608989891));
#72954=CARTESIAN_POINT('Ctrl Pts',(5.26413786481,-42.6372245963,2.77915560888));
#72955=CARTESIAN_POINT('Ctrl Pts',(5.20074359189,-42.5627311721,2.82109789633));
#72956=CARTESIAN_POINT('Ctrl Pts',(5.16924702152,-42.4684833924,2.84193758995));
#72957=CARTESIAN_POINT('Ctrl Pts',(5.16924702152,-42.3742356128,2.84193758995));
#72958=CARTESIAN_POINT('Ctrl Pts',(5.50717689409,-42.6742356128,2.86060629363));
#72959=CARTESIAN_POINT('Ctrl Pts',(5.41723711426,-42.6742356128,2.89155356331));
#72960=CARTESIAN_POINT('Ctrl Pts',(5.32729733443,-42.6372245963,2.92250083298));
#72961=CARTESIAN_POINT('Ctrl Pts',(5.25620894302,-42.5627311721,2.9469621888));
#72962=CARTESIAN_POINT('Ctrl Pts',(5.22088968328,-42.4684833924,2.95911451251));
#72963=CARTESIAN_POINT('Ctrl Pts',(5.22088968328,-42.3742356128,2.95911451251));
#72964=CARTESIAN_POINT('Ctrl Pts',(5.53155282798,-42.6742356128,2.94664996334));
#72965=CARTESIAN_POINT('Ctrl Pts',(5.43875945884,-42.6742356128,2.96752341897));
#72966=CARTESIAN_POINT('Ctrl Pts',(5.3459660897,-42.6372245963,2.9883968746));
#72967=CARTESIAN_POINT('Ctrl Pts',(5.27262225435,-42.5627311721,3.0048926648));
#72968=CARTESIAN_POINT('Ctrl Pts',(5.23618236028,-42.4684833924,3.0130922362));
#72969=CARTESIAN_POINT('Ctrl Pts',(5.23618236028,-42.3742356128,3.0130922362));
#72970=CARTESIAN_POINT('Ctrl Pts',(5.54384237615,-42.6742356128,3.03508099123));
#72971=CARTESIAN_POINT('Ctrl Pts',(5.44959461136,-42.6742356128,3.04553329529));
#72972=CARTESIAN_POINT('Ctrl Pts',(5.35534684657,-42.6372245963,3.05598559935));
#72973=CARTESIAN_POINT('Ctrl Pts',(5.28085341767,-42.5627311721,3.06424881978));
#72974=CARTESIAN_POINT('Ctrl Pts',(5.24384242331,-42.4684833924,3.06835170839));
#72975=CARTESIAN_POINT('Ctrl Pts',(5.24384242331,-42.3742356128,3.06835170839));
#72976=CARTESIAN_POINT('Ctrl Pts',(5.54384246963,-42.6742356128,3.12351053169));
#72977=CARTESIAN_POINT('Ctrl Pts',(5.44959469032,-42.6742356128,3.12351083782));
#72978=CARTESIAN_POINT('Ctrl Pts',(5.35534691101,-42.6372245963,3.12351114396));
#72979=CARTESIAN_POINT('Ctrl Pts',(5.28085348696,-42.5627311721,3.12351138593));
#72980=CARTESIAN_POINT('Ctrl Pts',(5.24384247058,-42.4684833924,3.12351150615));
#72981=CARTESIAN_POINT('Ctrl Pts',(5.24384247058,-42.3742356128,3.12351150615));
#72982=CARTESIAN_POINT('',(4.89234685374928,-42.3742356128,2.646074130721));
#72983=CARTESIAN_POINT('Origin',(4.980818894668,-42.3763569082249,2.36163710735502));
#72984=CARTESIAN_POINT('',(5.24384247076,-42.3742356128,3.12351150632));
#72985=CARTESIAN_POINT('Origin',(5.5417211288869,-42.3763569535561,3.1235105385842));
#72986=CARTESIAN_POINT('Ctrl Pts',(4.89234685393,-42.3742356128,2.64607413014));
#72987=CARTESIAN_POINT('Ctrl Pts',(5.01354316676,-42.3742356128,2.6837716054));
#72988=CARTESIAN_POINT('Ctrl Pts',(5.12322496214,-42.3742356128,2.76042445737));
#72989=CARTESIAN_POINT('Ctrl Pts',(5.20322505246,-42.3742356128,2.86908878029));
#72990=CARTESIAN_POINT('Ctrl Pts',(5.24384247076,-42.3742356128,2.9965877265));
#72991=CARTESIAN_POINT('Ctrl Pts',(5.24384247076,-42.3742356128,3.12351150632));
#72992=CARTESIAN_POINT('Ctrl Pts',(4.89234685393,-40.6742356128,2.64607413014));
#72993=CARTESIAN_POINT('Ctrl Pts',(4.89234685393,-42.7142356128,2.64607413014));
#72994=CARTESIAN_POINT('Ctrl Pts',(5.01354316676,-40.6742356128,2.6837716054));
#72995=CARTESIAN_POINT('Ctrl Pts',(5.01354316676,-42.7142356128,2.6837716054));
#72996=CARTESIAN_POINT('Ctrl Pts',(5.12322496214,-40.6742356128,2.76042445737));
#72997=CARTESIAN_POINT('Ctrl Pts',(5.12322496214,-42.7142356128,2.76042445737));
#72998=CARTESIAN_POINT('Ctrl Pts',(5.20322505246,-40.6742356128,2.86908878029));
#72999=CARTESIAN_POINT('Ctrl Pts',(5.20322505246,-42.7142356128,2.86908878029));
#73000=CARTESIAN_POINT('Ctrl Pts',(5.24384247076,-40.6742356128,2.9965877265));
#73001=CARTESIAN_POINT('Ctrl Pts',(5.24384247076,-42.7142356128,2.9965877265));
#73002=CARTESIAN_POINT('Ctrl Pts',(5.24384247076,-40.6742356128,3.12351150632));
#73003=CARTESIAN_POINT('Ctrl Pts',(5.24384247076,-42.7142356128,3.12351150632));
#73004=CARTESIAN_POINT('',(5.24384247076,-41.5242356128,3.12351150632));
#73005=CARTESIAN_POINT('',(4.89234685393,-41.6742356128,2.64607413014));
#73006=CARTESIAN_POINT('Origin',(5.54384247076,-42.3742356128,1.77756718468));
#73007=CARTESIAN_POINT('',(5.24384247076,-42.3742356128,6.92091964038719));
#73008=CARTESIAN_POINT('Origin',(5.54384247076,-42.3742356128,6.92091963994));
#73009=CARTESIAN_POINT('',(5.24384247076,-42.3742356128,5.02221557313));
#73010=CARTESIAN_POINT('Origin',(5.24384247076,-40.6742356128,3.12351150632));
#73011=CARTESIAN_POINT('',(5.24384247076,-41.6742356128,6.92091963994));
#73012=CARTESIAN_POINT('Ctrl Pts',(5.54384244762,-42.6742356128,6.92091961486));
#73013=CARTESIAN_POINT('Ctrl Pts',(5.44959466918,-42.6742356128,6.92091962424));
#73014=CARTESIAN_POINT('Ctrl Pts',(5.35534689074,-42.6372245963,6.92091963362));
#73015=CARTESIAN_POINT('Ctrl Pts',(5.28085346739,-42.5627311721,6.92091964103));
#73016=CARTESIAN_POINT('Ctrl Pts',(5.24384245134,-42.4684833924,6.92091964471));
#73017=CARTESIAN_POINT('Ctrl Pts',(5.24384245134,-42.3742356128,6.92091964471));
#73018=CARTESIAN_POINT('Ctrl Pts',(5.54384242174,-42.6742356128,7.79164279162));
#73019=CARTESIAN_POINT('Ctrl Pts',(5.44959464312,-42.6742356128,7.77690267016));
#73020=CARTESIAN_POINT('Ctrl Pts',(5.35534686449,-42.6372245963,7.76216254869));
#73021=CARTESIAN_POINT('Ctrl Pts',(5.28085344062,-42.5627311721,7.75051190074));
#73022=CARTESIAN_POINT('Ctrl Pts',(5.24384242488,-42.4684833924,7.74472352777));
#73023=CARTESIAN_POINT('Ctrl Pts',(5.24384242488,-42.3742356128,7.74472352777));
#73024=CARTESIAN_POINT('Ctrl Pts',(5.37333591464,-42.6742356128,8.66281176035));
#73025=CARTESIAN_POINT('Ctrl Pts',(5.28197913873,-42.6742356128,8.63316176369));
#73026=CARTESIAN_POINT('Ctrl Pts',(5.19062236283,-42.6372245963,8.60351176703));
#73027=CARTESIAN_POINT('Ctrl Pts',(5.11841398777,-42.5627311721,8.580076505));
#73028=CARTESIAN_POINT('Ctrl Pts',(5.08253826524,-42.4684833924,8.56843288973));
#73029=CARTESIAN_POINT('Ctrl Pts',(5.08253826524,-42.3742356128,8.56843288973));
#73030=CARTESIAN_POINT('Ctrl Pts',(5.03080493437,-42.6742356128,9.48834807329));
#73031=CARTESIAN_POINT('Ctrl Pts',(4.94530723737,-42.6742356128,9.44467844814));
#73032=CARTESIAN_POINT('Ctrl Pts',(4.85980954038,-42.6372245963,9.40100882299));
#73033=CARTESIAN_POINT('Ctrl Pts',(4.79223215539,-42.5627311721,9.36649233861));
#73034=CARTESIAN_POINT('Ctrl Pts',(4.75865731238,-42.4684833924,9.34934333918));
#73035=CARTESIAN_POINT('Ctrl Pts',(4.75865731238,-42.3742356128,9.34934333918));
#73036=CARTESIAN_POINT('Ctrl Pts',(4.04085177536,-42.6742356128,10.9614284297));
#73037=CARTESIAN_POINT('Ctrl Pts',(3.9721502684,-42.6742356128,10.8927236182));
#73038=CARTESIAN_POINT('Ctrl Pts',(3.90344876143,-42.6372245963,10.8240188068));
#73039=CARTESIAN_POINT('Ctrl Pts',(3.84914712943,-42.5627311721,10.7697145612));
#73040=CARTESIAN_POINT('Ctrl Pts',(3.82216808673,-42.4684833924,10.7427342225));
#73041=CARTESIAN_POINT('Ctrl Pts',(3.82216808673,-42.3742356128,10.7427342225));
#73042=CARTESIAN_POINT('Ctrl Pts',(2.56772513466,-42.6742356128,11.9513497364));
#73043=CARTESIAN_POINT('Ctrl Pts',(2.5240578489,-42.6742356128,11.8658510287));
#73044=CARTESIAN_POINT('Ctrl Pts',(2.48039056315,-42.6372245963,11.7803523209));
#73045=CARTESIAN_POINT('Ctrl Pts',(2.44587592617,-42.5627311721,11.7127741387));
#73046=CARTESIAN_POINT('Ctrl Pts',(2.42872784707,-42.4684833924,11.6791988971));
#73047=CARTESIAN_POINT('Ctrl Pts',(2.42872784707,-42.3742356128,11.6791988971));
#73048=CARTESIAN_POINT('Ctrl Pts',(1.74211448794,-42.6742356128,12.2938681423));
#73049=CARTESIAN_POINT('Ctrl Pts',(1.71247115576,-42.6742356128,12.2025094799));
#73050=CARTESIAN_POINT('Ctrl Pts',(1.68282782357,-42.6372245963,12.1111508175));
#73051=CARTESIAN_POINT('Ctrl Pts',(1.65939783581,-42.5627311721,12.0389409514));
#73052=CARTESIAN_POINT('Ctrl Pts',(1.647756831,-42.4684833924,12.003064488));
#73053=CARTESIAN_POINT('Ctrl Pts',(1.647756831,-42.3742356128,12.003064488));
#73054=CARTESIAN_POINT('Ctrl Pts',(0.870857634643,-42.6742356128,12.464345958));
#73055=CARTESIAN_POINT('Ctrl Pts',(0.856121049032,-42.6742356128,12.3700981819));
#73056=CARTESIAN_POINT('Ctrl Pts',(0.841384463421,-42.6372245963,12.2758504058));
#73057=CARTESIAN_POINT('Ctrl Pts',(0.829736605758,-42.5627311721,12.2013569839));
#73058=CARTESIAN_POINT('Ctrl Pts',(0.823949625757,-42.4684833924,12.1643459692));
#73059=CARTESIAN_POINT('Ctrl Pts',(0.823949625757,-42.3742356128,12.1643459692));
#73060=CARTESIAN_POINT('Ctrl Pts',(2.93507693705E-7,-42.6742356128,12.4643460018));
#73061=CARTESIAN_POINT('Ctrl Pts',(2.01415953693E-7,-42.6742356128,12.3700982223));
#73062=CARTESIAN_POINT('Ctrl Pts',(1.09324215014E-7,-42.6372245963,12.2758504427));
#73063=CARTESIAN_POINT('Ctrl Pts',(3.65349244191E-8,-42.5627311721,12.2013570185));
#73064=CARTESIAN_POINT('Ctrl Pts',(3.70582231568E-10,-42.4684833924,12.164346002));
#73065=CARTESIAN_POINT('Ctrl Pts',(3.70582675657E-10,-42.3742356128,12.164346002));
#73066=CARTESIAN_POINT('',(9.26471538767733E-11,-42.3742356128,12.1643460032));
#73067=CARTESIAN_POINT('Origin',(4.74561210871912E-7,-42.3763569069502,
12.4622247083968));
#73068=CARTESIAN_POINT('Ctrl Pts',(5.24384247076,-42.3742356128,6.92091963994));
#73069=CARTESIAN_POINT('Ctrl Pts',(5.24384247076,-42.3742356128,8.5681906143));
#73070=CARTESIAN_POINT('Ctrl Pts',(4.59882235543,-42.3742356128,10.2169985032));
#73071=CARTESIAN_POINT('Ctrl Pts',(3.29649497043,-42.3742356128,11.5193258882));
#73072=CARTESIAN_POINT('Ctrl Pts',(1.64768708151,-42.3742356128,12.1643460036));
#73073=CARTESIAN_POINT('Ctrl Pts',(3.10862446895E-15,-42.3742356128,12.1643460036));
#73074=CARTESIAN_POINT('Ctrl Pts',(5.24384247076,-40.6742356128,6.92091963994));
#73075=CARTESIAN_POINT('Ctrl Pts',(5.24384247076,-42.7142356128,6.92091963994));
#73076=CARTESIAN_POINT('Ctrl Pts',(5.24384247076,-40.6742356128,8.5681906143));
#73077=CARTESIAN_POINT('Ctrl Pts',(5.24384247076,-42.7142356128,8.5681906143));
#73078=CARTESIAN_POINT('Ctrl Pts',(4.59882235543,-40.6742356128,10.2169985032));
#73079=CARTESIAN_POINT('Ctrl Pts',(4.59882235543,-42.7142356128,10.2169985032));
#73080=CARTESIAN_POINT('Ctrl Pts',(3.29649497043,-40.6742356128,11.5193258882));
#73081=CARTESIAN_POINT('Ctrl Pts',(3.29649497043,-42.7142356128,11.5193258882));
#73082=CARTESIAN_POINT('Ctrl Pts',(1.64768708151,-40.6742356128,12.1643460036));
#73083=CARTESIAN_POINT('Ctrl Pts',(1.64768708151,-42.7142356128,12.1643460036));
#73084=CARTESIAN_POINT('Ctrl Pts',(1.66533453694E-15,-40.6742356128,12.1643460036));
#73085=CARTESIAN_POINT('Ctrl Pts',(1.66533453694E-15,-42.7142356128,12.1643460036));
#73086=CARTESIAN_POINT('',(1.7763568394E-15,-41.6742356128,12.1643460036));
#73087=CARTESIAN_POINT('Ctrl Pts',(2.6645352591E-15,-42.6742356128,12.4643460036));
#73088=CARTESIAN_POINT('Ctrl Pts',(2.6645352591E-15,-42.6742356128,12.3700982239));
#73089=CARTESIAN_POINT('Ctrl Pts',(3.99680288865E-15,-42.6372245963,12.2758504443));
#73090=CARTESIAN_POINT('Ctrl Pts',(3.99680288865E-15,-42.5627311721,12.2013570201));
#73091=CARTESIAN_POINT('Ctrl Pts',(3.5527136788E-15,-42.4684833924,12.1643460036));
#73092=CARTESIAN_POINT('Ctrl Pts',(3.5527136788E-15,-42.3742356128,12.1643460036));
#73093=CARTESIAN_POINT('Ctrl Pts',(-0.98432408905,-42.6742356128,12.4643460036));
#73094=CARTESIAN_POINT('Ctrl Pts',(-0.967642424377,-42.6742356128,12.3700982239));
#73095=CARTESIAN_POINT('Ctrl Pts',(-0.950960759704,-42.6372245963,12.2758504443));
#73096=CARTESIAN_POINT('Ctrl Pts',(-0.937775575531,-42.5627311721,12.20135702));
#73097=CARTESIAN_POINT('Ctrl Pts',(-0.931224701216,-42.4684833924,12.1643460036));
#73098=CARTESIAN_POINT('Ctrl Pts',(-0.931224701216,-42.3742356128,12.1643460036));
#73099=CARTESIAN_POINT('Ctrl Pts',(-1.96903536838,-42.6742356128,12.2466179469));
#73100=CARTESIAN_POINT('Ctrl Pts',(-1.9355445799,-42.6742356128,12.1560629127));
#73101=CARTESIAN_POINT('Ctrl Pts',(-1.90205379142,-42.6372245963,12.0655078786));
#73102=CARTESIAN_POINT('Ctrl Pts',(-1.87558267973,-42.5627311721,11.9939331994));
#73103=CARTESIAN_POINT('Ctrl Pts',(-1.86243087769,-42.4684833924,11.9583723207));
#73104=CARTESIAN_POINT('Ctrl Pts',(-1.86243087769,-42.3742356128,11.9583723207));
#73105=CARTESIAN_POINT('Ctrl Pts',(-2.88824914665,-42.6742356128,11.8085576616));
#73106=CARTESIAN_POINT('Ctrl Pts',(-2.83912141015,-42.6742356128,11.7255036705));
#73107=CARTESIAN_POINT('Ctrl Pts',(-2.78999367365,-42.6372245963,11.6424496795));
#73108=CARTESIAN_POINT('Ctrl Pts',(-2.75116312141,-42.5627311721,11.5768037983));
#73109=CARTESIAN_POINT('Ctrl Pts',(-2.7318707045,-42.4684833924,11.5441885971));
#73110=CARTESIAN_POINT('Ctrl Pts',(-2.7318707045,-42.3742356128,11.5441885971));
#73111=CARTESIAN_POINT('Ctrl Pts',(-4.2870492691,-42.6742356128,10.7016671976));
#73112=CARTESIAN_POINT('Ctrl Pts',(-4.214184775,-42.6742356128,10.6373567994));
#73113=CARTESIAN_POINT('Ctrl Pts',(-4.14132028091,-42.6372245963,10.5730464011));
#73114=CARTESIAN_POINT('Ctrl Pts',(-4.08372820096,-42.5627311721,10.5222154955));
#73115=CARTESIAN_POINT('Ctrl Pts',(-4.05511438087,-42.4684833924,10.4969608421));
#73116=CARTESIAN_POINT('Ctrl Pts',(-4.05511438087,-42.3742356128,10.4969608421));
#73117=CARTESIAN_POINT('Ctrl Pts',(-5.1560065879,-42.6742356128,9.16334308768));
#73118=CARTESIAN_POINT('Ctrl Pts',(-5.06836283571,-42.6742356128,9.12520886355));
#73119=CARTESIAN_POINT('Ctrl Pts',(-4.98071908353,-42.6372245963,9.08707463943));
#73120=CARTESIAN_POINT('Ctrl Pts',(-4.91144548089,-42.5627311721,9.05693334249));
#73121=CARTESIAN_POINT('Ctrl Pts',(-4.87702786008,-42.4684833924,9.04195808227));
#73122=CARTESIAN_POINT('Ctrl Pts',(-4.87702786008,-42.3742356128,9.04195808227));
#73123=CARTESIAN_POINT('Ctrl Pts',(-5.4148883553,-42.6742356128,8.4357571418));
#73124=CARTESIAN_POINT('Ctrl Pts',(-5.3228269536,-42.6742356128,8.40996790687));
#73125=CARTESIAN_POINT('Ctrl Pts',(-5.2307655519,-42.6372245963,8.38417867195));
#73126=CARTESIAN_POINT('Ctrl Pts',(-5.15800024067,-42.5627311721,8.36379492493));
#73127=CARTESIAN_POINT('Ctrl Pts',(-5.12184781233,-42.4684833924,8.35366745746));
#73128=CARTESIAN_POINT('Ctrl Pts',(-5.12184781233,-42.3742356128,8.35366745746));
#73129=CARTESIAN_POINT('Ctrl Pts',(-5.5438412969,-42.6742356128,7.67813852663));
#73130=CARTESIAN_POINT('Ctrl Pts',(-5.44959357541,-42.6742356128,7.66532863316));
#73131=CARTESIAN_POINT('Ctrl Pts',(-5.35534585392,-42.6372245963,7.65251873968));
#73132=CARTESIAN_POINT('Ctrl Pts',(-5.28085247527,-42.5627311721,7.64239376366));
#73133=CARTESIAN_POINT('Ctrl Pts',(-5.2438414819,-42.4684833924,7.6373633693));
#73134=CARTESIAN_POINT('Ctrl Pts',(-5.2438414819,-42.3742356128,7.6373633693));
#73135=CARTESIAN_POINT('Ctrl Pts',(-5.54384247523,-42.6742356128,6.92092019865));
#73136=CARTESIAN_POINT('Ctrl Pts',(-5.44959469539,-42.6742356128,6.92092002284));
#73137=CARTESIAN_POINT('Ctrl Pts',(-5.35534691555,-42.6372245963,6.92091984703));
#73138=CARTESIAN_POINT('Ctrl Pts',(-5.28085349108,-42.5627311721,6.92091970806));
#73139=CARTESIAN_POINT('Ctrl Pts',(-5.24384247449,-42.4684833924,6.92091963902));
#73140=CARTESIAN_POINT('Ctrl Pts',(-5.24384247449,-42.3742356128,6.92091963902));
#73141=CARTESIAN_POINT('',(-5.243842472625,-42.3742356128,6.92091963994));
#73142=CARTESIAN_POINT('Origin',(-5.54172113446363,-42.3763569535662,6.92092019624449));
#73143=CARTESIAN_POINT('Ctrl Pts',(2.94224766596691E-15,-42.3742356128,
12.1643460036));
#73144=CARTESIAN_POINT('Ctrl Pts',(-0.147449922720393,-42.3742356128,12.1643460036));
#73145=CARTESIAN_POINT('Ctrl Pts',(-0.294900815063498,-42.3742356128,12.1581447470062));
#73146=CARTESIAN_POINT('Ctrl Pts',(-0.441824896475511,-42.3742356128,12.145748963406));
#73147=CARTESIAN_POINT('Ctrl Pts',(-0.590135191421333,-42.3742356128,12.1332362268678));
#73148=CARTESIAN_POINT('Ctrl Pts',(-0.737908469878102,-42.3742356128,12.1144116091439));
#73149=CARTESIAN_POINT('Ctrl Pts',(-0.884608151694916,-42.3742356128,12.0893347773405));
#73150=CARTESIAN_POINT('Ctrl Pts',(-1.03930642893801,-42.3742356128,12.0628906662787));
#73151=CARTESIAN_POINT('Ctrl Pts',(-1.19281049201319,-42.3742356128,12.0294936516789));
#73152=CARTESIAN_POINT('Ctrl Pts',(-1.34450258526901,-42.3742356128,11.9892743993845));
#73153=CARTESIAN_POINT('Ctrl Pts',(-1.49136324514781,-42.3742356128,11.9503361409359));
#73154=CARTESIAN_POINT('Ctrl Pts',(-1.63652535204734,-42.3742356128,11.9050037934466));
#73155=CARTESIAN_POINT('Ctrl Pts',(-1.77944242181759,-42.3742356128,11.8534486481863));
#73156=CARTESIAN_POINT('Ctrl Pts',(-1.92321237006314,-42.3742356128,11.8015858400712));
#73157=CARTESIAN_POINT('Ctrl Pts',(-2.0647101495172,-42.3742356128,11.7434258871945));
#73158=CARTESIAN_POINT('Ctrl Pts',(-2.20339722846304,-42.3742356128,11.6791931653637));
#73159=CARTESIAN_POINT('Ctrl Pts',(-2.34273810420776,-42.3742356128,11.6146576384826));
#73160=CARTESIAN_POINT('Ctrl Pts',(-2.479241454579,-42.3742356128,11.543992114104));
#73161=CARTESIAN_POINT('Ctrl Pts',(-2.61238291383962,-42.3742356128,11.4674721362935));
#73162=CARTESIAN_POINT('Ctrl Pts',(-2.75114825234043,-42.3742356128,11.3877199638153));
#73163=CARTESIAN_POINT('Ctrl Pts',(-2.88626120444508,-42.3742356128,11.3016081914638));
#73164=CARTESIAN_POINT('Ctrl Pts',(-3.01715771894491,-42.3742356128,11.2095008346905));
#73165=CARTESIAN_POINT('Ctrl Pts',(-3.1434013231585,-42.3742356128,11.1206675701983));
#73166=CARTESIAN_POINT('Ctrl Pts',(-3.26572284156763,-42.3742356128,11.026257876475));
#73167=CARTESIAN_POINT('Ctrl Pts',(-3.38364680560608,-42.3742356128,10.9266419252746));
#73168=CARTESIAN_POINT('Ctrl Pts',(-3.50150366185979,-42.3742356128,10.8270826631947));
#73169=CARTESIAN_POINT('Ctrl Pts',(-3.61496771838722,-42.3742356128,10.7223232785427));
#73170=CARTESIAN_POINT('Ctrl Pts',(-3.72359807694681,-42.3742356128,10.6127729063755));
#73171=CARTESIAN_POINT('Ctrl Pts',(-3.83193116474364,-42.3742356128,10.5035223226202));
#73172=CARTESIAN_POINT('Ctrl Pts',(-3.93545674116179,-42.3742356128,10.3895071587474));
#73173=CARTESIAN_POINT('Ctrl Pts',(-4.03377468497118,-42.3742356128,10.271169329208));
#73174=CARTESIAN_POINT('Ctrl Pts',(-4.04506377902863,-42.3742356128,10.2575815054959));
#73175=CARTESIAN_POINT('Ctrl Pts',(-4.05628425744536,-42.3742356128,10.2439367281876));
#73176=CARTESIAN_POINT('Ctrl Pts',(-4.06743554813384,-42.3742356128,10.2302356948108));
#73177=CARTESIAN_POINT('Ctrl Pts',(-4.16409419458107,-42.3742356128,10.1114760482251));
#73178=CARTESIAN_POINT('Ctrl Pts',(-4.25555110734879,-42.3742356128,9.98848713576328));
#73179=CARTESIAN_POINT('Ctrl Pts',(-4.34145194270822,-42.3742356128,9.86173891404879));
#73180=CARTESIAN_POINT('Ctrl Pts',(-4.42735924310164,-42.3742356128,9.73498115306081));
#73181=CARTESIAN_POINT('Ctrl Pts',(-4.50770946494624,-42.3742356128,9.60446378646192));
#73182=CARTESIAN_POINT('Ctrl Pts',(-4.58219157674198,-42.3742356128,9.47068578032751));
#73183=CARTESIAN_POINT('Ctrl Pts',(-4.65656344968784,-42.3742356128,9.33710577520543));
#73184=CARTESIAN_POINT('Ctrl Pts',(-4.72508441832579,-42.3742356128,9.20027505005788));
#73185=CARTESIAN_POINT('Ctrl Pts',(-4.78749044755381,-42.3742356128,9.06071508722799));
#73186=CARTESIAN_POINT('Ctrl Pts',(-4.84971102952993,-42.3742356128,8.92156984412792));
#73187=CARTESIAN_POINT('Ctrl Pts',(-4.90585282355185,-42.3742356128,8.77971183518736));
#73188=CARTESIAN_POINT('Ctrl Pts',(-4.9557016653129,-42.3742356128,8.63567838517432));
#73189=CARTESIAN_POINT('Ctrl Pts',(-5.00519016121833,-42.3742356128,8.49268611997015));
#73190=CARTESIAN_POINT('Ctrl Pts',(-5.04847625992148,-42.3742356128,8.3475500284784));
#73191=CARTESIAN_POINT('Ctrl Pts',(-5.085399006776,-42.3742356128,8.20081194497571));
#73192=CARTESIAN_POINT('Ctrl Pts',(-5.12213010100009,-42.3742356128,8.05483552581506));
#73193=CARTESIAN_POINT('Ctrl Pts',(-5.15256362407304,-42.3742356128,7.90727396260646));
#73194=CARTESIAN_POINT('Ctrl Pts',(-5.17659093071025,-42.3742356128,7.75867267407153));
#73195=CARTESIAN_POINT('Ctrl Pts',(-5.20038237069215,-42.3742356128,7.61153014616394));
#73196=CARTESIAN_POINT('Ctrl Pts',(-5.2178926901178,-42.3742356128,7.46336845857782));
#73197=CARTESIAN_POINT('Ctrl Pts',(-5.22906657671221,-42.3742356128,7.31472507751491));
#73198=CARTESIAN_POINT('Ctrl Pts',(-5.23891552865557,-42.3742356128,7.18370696627698));
#73199=CARTESIAN_POINT('Ctrl Pts',(-5.24384229242681,-42.3742356128,7.05231483928685));
#73200=CARTESIAN_POINT('Ctrl Pts',(-5.24384247449,-42.3742356128,6.92091963994));
#73201=CARTESIAN_POINT('Ctrl Pts',(1.55431223448E-15,-40.6742356128,12.1643460036));
#73202=CARTESIAN_POINT('Ctrl Pts',(1.55431223448E-15,-42.7142356128,12.1643460036));
#73203=CARTESIAN_POINT('Ctrl Pts',(-1.64768708151,-40.6742356128,12.1643460036));
#73204=CARTESIAN_POINT('Ctrl Pts',(-1.64768708151,-42.7142356128,12.1643460036));
#73205=CARTESIAN_POINT('Ctrl Pts',(-3.29649497043,-40.6742356128,11.5193258882));
#73206=CARTESIAN_POINT('Ctrl Pts',(-3.29649497043,-42.7142356128,11.5193258882));
#73207=CARTESIAN_POINT('Ctrl Pts',(-4.59882235543,-40.6742356128,10.2169985032));
#73208=CARTESIAN_POINT('Ctrl Pts',(-4.59882235543,-42.7142356128,10.2169985032));
#73209=CARTESIAN_POINT('Ctrl Pts',(-5.24384247076,-40.6742356128,8.5681906143));
#73210=CARTESIAN_POINT('Ctrl Pts',(-5.24384247076,-42.7142356128,8.5681906143));
#73211=CARTESIAN_POINT('Ctrl Pts',(-5.24384247076,-40.6742356128,6.92091963994));
#73212=CARTESIAN_POINT('Ctrl Pts',(-5.24384247076,-42.7142356128,6.92091963994));
#73213=CARTESIAN_POINT('',(-5.24384247076,-41.5242356128,6.92091963994));
#73214=CARTESIAN_POINT('Origin',(-5.54384247076,-42.3742356128,1.77756718468));
#73215=CARTESIAN_POINT('',(-5.24384247076,-42.3742356128,3.12351150632));
#73216=CARTESIAN_POINT('Origin',(-5.54172117965729,-42.3763569039027,3.12351150632264));
#73217=CARTESIAN_POINT('',(-5.24384247076,-42.3742356128,5.02221557313));
#73218=CARTESIAN_POINT('Origin',(-5.24384247076,-40.6742356128,6.92091963994));
#73219=CARTESIAN_POINT('',(-5.24384247076,-41.6742356128,3.12351150632));
#73220=CARTESIAN_POINT('Ctrl Pts',(-5.54384247076,-42.6742356128,3.12351150632));
#73221=CARTESIAN_POINT('Ctrl Pts',(-5.44959469115,-42.6742356128,3.12351150632));
#73222=CARTESIAN_POINT('Ctrl Pts',(-5.35534691154,-42.6372245963,3.12351150632));
#73223=CARTESIAN_POINT('Ctrl Pts',(-5.28085348726,-42.5627311721,3.12351150632));
#73224=CARTESIAN_POINT('Ctrl Pts',(-5.24384247076,-42.4684833924,3.12351150632));
#73225=CARTESIAN_POINT('Ctrl Pts',(-5.24384247076,-42.3742356128,3.12351150632));
#73226=CARTESIAN_POINT('Ctrl Pts',(-5.54384247076,-42.6742356128,3.00871019694));
#73227=CARTESIAN_POINT('Ctrl Pts',(-5.44959469115,-42.6742356128,3.02230673235));
#73228=CARTESIAN_POINT('Ctrl Pts',(-5.35534691154,-42.6372245963,3.03590326776));
#73229=CARTESIAN_POINT('Ctrl Pts',(-5.28085348822,-42.5627311721,3.04664996844));
#73230=CARTESIAN_POINT('Ctrl Pts',(-5.24384247076,-42.4684833924,3.05198931333));
#73231=CARTESIAN_POINT('Ctrl Pts',(-5.24384247076,-42.3742356128,3.05198931333));
#73232=CARTESIAN_POINT('Ctrl Pts',(-5.52315912182,-42.6742356128,2.89410223843));
#73233=CARTESIAN_POINT('Ctrl Pts',(-5.43135552331,-42.6742356128,2.9210945322));
#73234=CARTESIAN_POINT('Ctrl Pts',(-5.3395519248,-42.6372245963,2.94808682596));
#73235=CARTESIAN_POINT('Ctrl Pts',(-5.26699037711,-42.5627311721,2.9694215235));
#73236=CARTESIAN_POINT('Ctrl Pts',(-5.23093919189,-42.4684833924,2.980021378));
#73237=CARTESIAN_POINT('Ctrl Pts',(-5.23093919189,-42.3742356128,2.980021378));
#73238=CARTESIAN_POINT('Ctrl Pts',(-5.48214276556,-42.6742356128,2.78431808342));
#73239=CARTESIAN_POINT('Ctrl Pts',(-5.39515201423,-42.6742356128,2.82425482107));
#73240=CARTESIAN_POINT('Ctrl Pts',(-5.30816126289,-42.6372245963,2.86419155871));
#73241=CARTESIAN_POINT('Ctrl Pts',(-5.23940274386,-42.5627311721,2.89575722697));
#73242=CARTESIAN_POINT('Ctrl Pts',(-5.205242604,-42.4684833924,2.91144066757));
#73243=CARTESIAN_POINT('Ctrl Pts',(-5.205242604,-42.3742356128,2.91144066757));
#73244=CARTESIAN_POINT('Ctrl Pts',(-5.3761771061,-42.6742356128,2.60732114997));
#73245=CARTESIAN_POINT('Ctrl Pts',(-5.30168431114,-42.6742356128,2.66814622051));
#73246=CARTESIAN_POINT('Ctrl Pts',(-5.22719151618,-42.6372245963,2.72897129106));
#73247=CARTESIAN_POINT('Ctrl Pts',(-5.16831323005,-42.5627311721,2.77704765466));
#73248=CARTESIAN_POINT('Ctrl Pts',(-5.13905917525,-42.4684833924,2.80093336279));
#73249=CARTESIAN_POINT('Ctrl Pts',(-5.13905917525,-42.3742356128,2.80093336279));
#73250=CARTESIAN_POINT('Ctrl Pts',(-5.221601036,-42.6742356128,2.47270789076));
#73251=CARTESIAN_POINT('Ctrl Pts',(-5.16533736648,-42.6742356128,2.54939750536));
#73252=CARTESIAN_POINT('Ctrl Pts',(-5.10907369696,-42.6372245963,2.62608711997));
#73253=CARTESIAN_POINT('Ctrl Pts',(-5.06460229045,-42.5627311721,2.686702393));
#73254=CARTESIAN_POINT('Ctrl Pts',(-5.04250821359,-42.4684833924,2.71681851572));
#73255=CARTESIAN_POINT('Ctrl Pts',(-5.04250821359,-42.3742356128,2.71681851572));
#73256=CARTESIAN_POINT('Ctrl Pts',(-5.14667997426,-42.6742356128,2.42387620273));
#73257=CARTESIAN_POINT('Ctrl Pts',(-5.09918799439,-42.6742356128,2.5062826488));
#73258=CARTESIAN_POINT('Ctrl Pts',(-5.05169601452,-42.6372245963,2.58868909488));
#73259=CARTESIAN_POINT('Ctrl Pts',(-5.01416083888,-42.5627311721,2.6538238772));
#73260=CARTESIAN_POINT('Ctrl Pts',(-4.99550830718,-42.4684833924,2.68618406744));
#73261=CARTESIAN_POINT('Ctrl Pts',(-4.99550830718,-42.3742356128,2.68618406744));
#73262=CARTESIAN_POINT('Ctrl Pts',(-5.06588952194,-42.6742356128,2.38587643296));
#73263=CARTESIAN_POINT('Ctrl Pts',(-5.02791646833,-42.6742356128,2.47276681809));
#73264=CARTESIAN_POINT('Ctrl Pts',(-4.98994341473,-42.6372245963,2.55965720322));
#73265=CARTESIAN_POINT('Ctrl Pts',(-4.95992787275,-42.5627311721,2.62833484879));
#73266=CARTESIAN_POINT('Ctrl Pts',(-4.94501753823,-42.4684833924,2.66245711898));
#73267=CARTESIAN_POINT('Ctrl Pts',(-4.94501753823,-42.3742356128,2.66245711898));
#73268=CARTESIAN_POINT('Ctrl Pts',(-4.98145041415,-42.6742356128,2.35961199498));
#73269=CARTESIAN_POINT('Ctrl Pts',(-4.95345770517,-42.6742356128,2.44960672899));
#73270=CARTESIAN_POINT('Ctrl Pts',(-4.92546499618,-42.6372245963,2.53960146299));
#73271=CARTESIAN_POINT('Ctrl Pts',(-4.90333956515,-42.5627311721,2.61073328096));
#73272=CARTESIAN_POINT('Ctrl Pts',(-4.89234685404,-42.4684833924,2.64607413036));
#73273=CARTESIAN_POINT('Ctrl Pts',(-4.89234685404,-42.3742356128,2.64607413036));
#73274=CARTESIAN_POINT('',(-4.89234685393,-42.3742356128,2.64607413014));
#73275=CARTESIAN_POINT('Origin',(-4.98082094568694,-42.3763569061133,2.36163774248594));
#73276=CARTESIAN_POINT('Ctrl Pts',(-5.24384247076,-42.3742356128,3.12351150632));
#73277=CARTESIAN_POINT('Ctrl Pts',(-5.24384247076,-42.3742356128,2.9965877265));
#73278=CARTESIAN_POINT('Ctrl Pts',(-5.20322505246,-42.3742356128,2.86908878029));
#73279=CARTESIAN_POINT('Ctrl Pts',(-5.12322496214,-42.3742356128,2.76042445737));
#73280=CARTESIAN_POINT('Ctrl Pts',(-5.01354316676,-42.3742356128,2.6837716054));
#73281=CARTESIAN_POINT('Ctrl Pts',(-4.89234685393,-42.3742356128,2.64607413014));
#73282=CARTESIAN_POINT('Ctrl Pts',(-5.24384247076,-40.6742356128,3.12351150632));
#73283=CARTESIAN_POINT('Ctrl Pts',(-5.24384247076,-42.7142356128,3.12351150632));
#73284=CARTESIAN_POINT('Ctrl Pts',(-5.24384247076,-40.6742356128,2.9965877265));
#73285=CARTESIAN_POINT('Ctrl Pts',(-5.24384247076,-42.7142356128,2.9965877265));
#73286=CARTESIAN_POINT('Ctrl Pts',(-5.20322505246,-40.6742356128,2.86908878029));
#73287=CARTESIAN_POINT('Ctrl Pts',(-5.20322505246,-42.7142356128,2.86908878029));
#73288=CARTESIAN_POINT('Ctrl Pts',(-5.12322496214,-40.6742356128,2.76042445737));
#73289=CARTESIAN_POINT('Ctrl Pts',(-5.12322496214,-42.7142356128,2.76042445737));
#73290=CARTESIAN_POINT('Ctrl Pts',(-5.01354316676,-40.6742356128,2.6837716054));
#73291=CARTESIAN_POINT('Ctrl Pts',(-5.01354316676,-42.7142356128,2.6837716054));
#73292=CARTESIAN_POINT('Ctrl Pts',(-4.89234685393,-40.6742356128,2.64607413014));
#73293=CARTESIAN_POINT('Ctrl Pts',(-4.89234685393,-42.7142356128,2.64607413014));
#73294=CARTESIAN_POINT('',(-4.89234685393,-41.6742356128,2.64607413014));
#73295=CARTESIAN_POINT('Ctrl Pts',(-4.98144948383,-42.6742356128,2.35961170443));
#73296=CARTESIAN_POINT('Ctrl Pts',(-4.95345706708,-42.6742356128,2.44960652964));
#73297=CARTESIAN_POINT('Ctrl Pts',(-4.92546465033,-42.6372245963,2.53960135485));
#73298=CARTESIAN_POINT('Ctrl Pts',(-4.90333945028,-42.5627311721,2.61073324492));
#73299=CARTESIAN_POINT('Ctrl Pts',(-4.89234685393,-42.4684833924,2.64607413014));
#73300=CARTESIAN_POINT('Ctrl Pts',(-4.89234685393,-42.3742356128,2.64607413014));
#73301=CARTESIAN_POINT('Ctrl Pts',(-4.28684551132,-42.6742356128,2.14355879439));
#73302=CARTESIAN_POINT('Ctrl Pts',(-4.24825002553,-42.6742356128,2.23025559078));
#73303=CARTESIAN_POINT('Ctrl Pts',(-4.20965453974,-42.6372245963,2.31695238717));
#73304=CARTESIAN_POINT('Ctrl Pts',(-4.17914867624,-42.5627311721,2.38547751597));
#73305=CARTESIAN_POINT('Ctrl Pts',(-4.16399226443,-42.4684833924,2.41952326831));
#73306=CARTESIAN_POINT('Ctrl Pts',(-4.16399226443,-42.3742356128,2.41952326831));
#73307=CARTESIAN_POINT('Ctrl Pts',(-3.62343950079,-42.6742356128,1.82501616557));
#73308=CARTESIAN_POINT('Ctrl Pts',(-3.57482509928,-42.6742356128,1.90688399481));
#73309=CARTESIAN_POINT('Ctrl Pts',(-3.52621069777,-42.6372245963,1.98875182405));
#73310=CARTESIAN_POINT('Ctrl Pts',(-3.48778588555,-42.5627311721,2.05346013832));
#73311=CARTESIAN_POINT('Ctrl Pts',(-3.46869505468,-42.4684833924,2.08560955965));
#73312=CARTESIAN_POINT('Ctrl Pts',(-3.46869505468,-42.3742356128,2.08560955965));
#73313=CARTESIAN_POINT('Ctrl Pts',(-3.01239604925,-42.6742356128,1.41174509036));
#73314=CARTESIAN_POINT('Ctrl Pts',(-2.95448305204,-42.6742356128,1.48733455128));
#73315=CARTESIAN_POINT('Ctrl Pts',(-2.89657005483,-42.6372245963,1.5629240122));
#73316=CARTESIAN_POINT('Ctrl Pts',(-2.85079564102,-42.5627311721,1.62266993413));
#73317=CARTESIAN_POINT('Ctrl Pts',(-2.82805325375,-42.4684833924,1.65235381737));
#73318=CARTESIAN_POINT('Ctrl Pts',(-2.82805325375,-42.3742356128,1.65235381737));
#73319=CARTESIAN_POINT('Ctrl Pts',(-2.04894527302,-42.6742356128,0.527537333153));
#73320=CARTESIAN_POINT('Ctrl Pts',(-1.97636933137,-42.6742356128,0.589684852453));
#73321=CARTESIAN_POINT('Ctrl Pts',(-1.90379338972,-42.6372245963,0.651832371753));
#73322=CARTESIAN_POINT('Ctrl Pts',(-1.84642937642,-42.5627311721,0.700953735078));
#73323=CARTESIAN_POINT('Ctrl Pts',(-1.81792887576,-42.4684833924,0.725359031103));
#73324=CARTESIAN_POINT('Ctrl Pts',(-1.81792887576,-42.3742356128,0.725359031103));
#73325=CARTESIAN_POINT('Ctrl Pts',(-1.34746460805,-42.6742356128,-0.569990686554));
#73326=CARTESIAN_POINT('Ctrl Pts',(-1.26422030149,-42.6742356128,-0.524548982088));
#73327=CARTESIAN_POINT('Ctrl Pts',(-1.18097599493,-42.6372245963,-0.479107277622));
#73328=CARTESIAN_POINT('Ctrl Pts',(-1.11517971718,-42.5627311721,-0.443190147097));
#73329=CARTESIAN_POINT('Ctrl Pts',(-1.08248975058,-42.4684833924,-0.425345248789));
#73330=CARTESIAN_POINT('Ctrl Pts',(-1.08248975058,-42.3742356128,-0.425345248789));
#73331=CARTESIAN_POINT('Ctrl Pts',(-1.09663661983,-42.6742356128,-1.08402978875));
#73332=CARTESIAN_POINT('Ctrl Pts',(-1.00960204779,-42.6742356128,-1.04634891047));
#73333=CARTESIAN_POINT('Ctrl Pts',(-0.92256747575,-42.6372245963,-1.0086680322));
#73334=CARTESIAN_POINT('Ctrl Pts',(-0.853775353599,-42.5627311721,-0.978885143705));
#73335=CARTESIAN_POINT('Ctrl Pts',(-0.81959697263,-42.4684833924,-0.964087827993));
#73336=CARTESIAN_POINT('Ctrl Pts',(-0.81959697263,-42.3742356128,-0.964087827993));
#73337=CARTESIAN_POINT('Ctrl Pts',(-0.906464192514,-42.6742356128,-1.62228962869));
#73338=CARTESIAN_POINT('Ctrl Pts',(-0.816530141078,-42.6742356128,-1.59281044263));
#73339=CARTESIAN_POINT('Ctrl Pts',(-0.726596089643,-42.6372245963,-1.56333125657));
#73340=CARTESIAN_POINT('Ctrl Pts',(-0.655512245516,-42.5627311721,-1.54003086813));
#73341=CARTESIAN_POINT('Ctrl Pts',(-0.620195215749,-42.4684833924,-1.52845446509));
#73342=CARTESIAN_POINT('Ctrl Pts',(-0.620195215749,-42.3742356128,-1.52845446509));
#73343=CARTESIAN_POINT('Ctrl Pts',(-0.779760514736,-42.6742356128,-2.17481998786));
#73344=CARTESIAN_POINT('Ctrl Pts',(-0.68789712753,-42.6742356128,-2.15375432708));
#73345=CARTESIAN_POINT('Ctrl Pts',(-0.596033740324,-42.6372245963,-2.13268866631));
#73346=CARTESIAN_POINT('Ctrl Pts',(-0.523424939273,-42.5627311721,-2.11603837266));
#73347=CARTESIAN_POINT('Ctrl Pts',(-0.487350271475,-42.4684833924,-2.10776590702));
#73348=CARTESIAN_POINT('Ctrl Pts',(-0.487350271475,-42.3742356128,-2.10776590702));
#73349=CARTESIAN_POINT('',(-0.487350273345822,-42.3742356128,-2.10776590704375));
#73350=CARTESIAN_POINT('Origin',(-0.777692936443982,-42.3763569081971,-2.17434563581814));
#73351=CARTESIAN_POINT('Ctrl Pts',(-4.89234685393,-42.3742356128,2.64607413014));
#73352=CARTESIAN_POINT('Ctrl Pts',(-3.59661572838,-42.3742356128,2.2430437828));
#73353=CARTESIAN_POINT('Ctrl Pts',(-2.40362850687,-42.3742356128,1.49964984368));
#73354=CARTESIAN_POINT('Ctrl Pts',(-1.44114622406,-42.3742356128,0.46094601538));
#73355=CARTESIAN_POINT('Ctrl Pts',(-0.790651846747,-42.3742356128,-0.785131881257));
#73356=CARTESIAN_POINT('Ctrl Pts',(-0.48735027394,-42.3742356128,-2.10776590718));
#73357=CARTESIAN_POINT('Ctrl Pts',(-4.89234685393,-40.6742356128,2.64607413014));
#73358=CARTESIAN_POINT('Ctrl Pts',(-4.89234685393,-42.7142356128,2.64607413014));
#73359=CARTESIAN_POINT('Ctrl Pts',(-3.59661572838,-40.6742356128,2.2430437828));
#73360=CARTESIAN_POINT('Ctrl Pts',(-3.59661572838,-42.7142356128,2.2430437828));
#73361=CARTESIAN_POINT('Ctrl Pts',(-2.40362850687,-40.6742356128,1.49964984368));
#73362=CARTESIAN_POINT('Ctrl Pts',(-2.40362850687,-42.7142356128,1.49964984368));
#73363=CARTESIAN_POINT('Ctrl Pts',(-1.44114622406,-40.6742356128,0.46094601538));
#73364=CARTESIAN_POINT('Ctrl Pts',(-1.44114622406,-42.7142356128,0.46094601538));
#73365=CARTESIAN_POINT('Ctrl Pts',(-0.790651846747,-40.6742356128,-0.785131881257));
#73366=CARTESIAN_POINT('Ctrl Pts',(-0.790651846747,-42.7142356128,-0.785131881257));
#73367=CARTESIAN_POINT('Ctrl Pts',(-0.48735027394,-40.6742356128,-2.10776590718));
#73368=CARTESIAN_POINT('Ctrl Pts',(-0.48735027394,-42.7142356128,-2.10776590718));
#73369=CARTESIAN_POINT('',(-0.48735027394,-41.6742356128,-2.10776590718));
#73370=CARTESIAN_POINT('Ctrl Pts',(-0.779760438305,-42.6742356128,-2.17482033117));
#73371=CARTESIAN_POINT('Ctrl Pts',(-0.687897075884,-42.6742356128,-2.15375456259));
#73372=CARTESIAN_POINT('Ctrl Pts',(-0.596033713464,-42.6372245963,-2.13268879401));
#73373=CARTESIAN_POINT('Ctrl Pts',(-0.523424932005,-42.5627311721,-2.11603841516));
#73374=CARTESIAN_POINT('Ctrl Pts',(-0.48735027394,-42.4684833924,-2.10776590718));
#73375=CARTESIAN_POINT('Ctrl Pts',(-0.48735027394,-42.3742356128,-2.10776590718));
#73376=CARTESIAN_POINT('Ctrl Pts',(-0.728940682779,-42.6742356128,-2.39643453918));
#73377=CARTESIAN_POINT('Ctrl Pts',(-0.643021055832,-42.6742356128,-2.34944939701));
#73378=CARTESIAN_POINT('Ctrl Pts',(-0.557101428885,-42.6372245963,-2.30246425483));
#73379=CARTESIAN_POINT('Ctrl Pts',(-0.489190575517,-42.5627311721,-2.26532720315));
#73380=CARTESIAN_POINT('Ctrl Pts',(-0.455450016034,-42.4684833924,-2.2468761866));
#73381=CARTESIAN_POINT('Ctrl Pts',(-0.455450016034,-42.3742356128,-2.2468761866));
#73382=CARTESIAN_POINT('Ctrl Pts',(-0.600115266646,-42.6742356128,-2.60147317882));
#73383=CARTESIAN_POINT('Ctrl Pts',(-0.529241757754,-42.6742356128,-2.53022408265));
#73384=CARTESIAN_POINT('Ctrl Pts',(-0.458368248863,-42.6372245963,-2.45897498649));
#73385=CARTESIAN_POINT('Ctrl Pts',(-0.402349836567,-42.5627311721,-2.40265972476));
#73386=CARTESIAN_POINT('Ctrl Pts',(-0.374517881159,-42.4684833924,-2.3746802619));
#73387=CARTESIAN_POINT('Ctrl Pts',(-0.374517881159,-42.3742356128,-2.3746802619));
#73388=CARTESIAN_POINT('Ctrl Pts',(-0.397739638795,-42.6742356128,-2.74850259847));
#73389=CARTESIAN_POINT('Ctrl Pts',(-0.35125139287,-42.6742356128,-2.65967101811));
#73390=CARTESIAN_POINT('Ctrl Pts',(-0.304763146945,-42.6372245963,-2.57083943775));
#73391=CARTESIAN_POINT('Ctrl Pts',(-0.26801875295,-42.5627311721,-2.50062658719));
#73392=CARTESIAN_POINT('Ctrl Pts',(-0.249762956102,-42.4684833924,-2.46574289613));
#73393=CARTESIAN_POINT('Ctrl Pts',(-0.249762956102,-42.3742356128,-2.46574289613));
#73394=CARTESIAN_POINT('Ctrl Pts',(0.0424568072293,-42.6742356128,-2.86620382326));
#73395=CARTESIAN_POINT('Ctrl Pts',(0.0375764440826,-42.6742356128,-2.76378874984));
#73396=CARTESIAN_POINT('Ctrl Pts',(0.0326960809359,-42.6372245963,-2.66137367642));
#73397=CARTESIAN_POINT('Ctrl Pts',(0.0288385715632,-42.5627311721,-2.58042517097));
#73398=CARTESIAN_POINT('Ctrl Pts',(0.0269221288516,-42.4684833924,-2.54020651962));
#73399=CARTESIAN_POINT('Ctrl Pts',(0.0269221288516,-42.3742356128,-2.54020651962));
#73400=CARTESIAN_POINT('Ctrl Pts',(0.461136763067,-42.6742356128,-2.69888825006));
#73401=CARTESIAN_POINT('Ctrl Pts',(0.407040904949,-42.6742356128,-2.61589041711));
#73402=CARTESIAN_POINT('Ctrl Pts',(0.35294504683,-42.6372245963,-2.53289258416));
#73403=CARTESIAN_POINT('Ctrl Pts',(0.310187744589,-42.5627311721,-2.46729080736));
#73404=CARTESIAN_POINT('Ctrl Pts',(0.288944298659,-42.4684833924,-2.43469794247));
#73405=CARTESIAN_POINT('Ctrl Pts',(0.288944298659,-42.3742356128,-2.43469794247));
#73406=CARTESIAN_POINT('Ctrl Pts',(0.6271830499,-42.6742356128,-2.55661546807));
#73407=CARTESIAN_POINT('Ctrl Pts',(0.553146114073,-42.6742356128,-2.49065409452));
#73408=CARTESIAN_POINT('Ctrl Pts',(0.479109178246,-42.6372245963,-2.42469272097));
#73409=CARTESIAN_POINT('Ctrl Pts',(0.420590142213,-42.5627311721,-2.37255809298));
#73410=CARTESIAN_POINT('Ctrl Pts',(0.391516163736,-42.4684833924,-2.346653895));
#73411=CARTESIAN_POINT('Ctrl Pts',(0.391516163736,-42.3742356128,-2.346653895));
#73412=CARTESIAN_POINT('Ctrl Pts',(0.734479238607,-42.6742356128,-2.37228010264));
#73413=CARTESIAN_POINT('Ctrl Pts',(0.647901224488,-42.6742356128,-2.3281663573));
#73414=CARTESIAN_POINT('Ctrl Pts',(0.561323210368,-42.6372245963,-2.28405261197));
#73415=CARTESIAN_POINT('Ctrl Pts',(0.492892136152,-42.5627311721,-2.2491842994));
#73416=CARTESIAN_POINT('Ctrl Pts',(0.458892860404,-42.4684833924,-2.23186169008));
#73417=CARTESIAN_POINT('Ctrl Pts',(0.458892860404,-42.3742356128,-2.23186169008));
#73418=CARTESIAN_POINT('Ctrl Pts',(0.77975997749,-42.6742356128,-2.17482231881));
#73419=CARTESIAN_POINT('Ctrl Pts',(0.687896759445,-42.6742356128,-2.15375592622));
#73420=CARTESIAN_POINT('Ctrl Pts',(0.596033541399,-42.6372245963,-2.13268953362));
#73421=CARTESIAN_POINT('Ctrl Pts',(0.523424874053,-42.5627311721,-2.11603866155));
#73422=CARTESIAN_POINT('Ctrl Pts',(0.487350272685,-42.4684833924,-2.10776590852));
#73423=CARTESIAN_POINT('Ctrl Pts',(0.487350272685,-42.3742356128,-2.10776590852));
#73424=CARTESIAN_POINT('',(0.48735027362625,-42.3742356128,-2.107765907515));
#73425=CARTESIAN_POINT('Origin',(0.777692065618351,-42.3763569132498,-2.17434940414811));
#73426=CARTESIAN_POINT('Ctrl Pts',(-0.48735027394,-42.3742356128,-2.10776590718));
#73427=CARTESIAN_POINT('Ctrl Pts',(-0.481651530051025,-42.3742356128,-2.13261692428069));
#73428=CARTESIAN_POINT('Ctrl Pts',(-0.474067950247163,-42.3742356128,-2.15704737654675));
#73429=CARTESIAN_POINT('Ctrl Pts',(-0.46468020372962,-42.3742356128,-2.18075399603358));
#73430=CARTESIAN_POINT('Ctrl Pts',(-0.454943458649678,-42.3742356128,-2.20534193204347));
#73431=CARTESIAN_POINT('Ctrl Pts',(-0.443265892704172,-42.3742356128,-2.22915084671963));
#73432=CARTESIAN_POINT('Ctrl Pts',(-0.429786360652213,-42.3742356128,-2.25187433028169));
#73433=CARTESIAN_POINT('Ctrl Pts',(-0.416540327134175,-42.3742356128,-2.27420418741245));
#73434=CARTESIAN_POINT('Ctrl Pts',(-0.40155462641195,-42.3742356128,-2.29548581661124));
#73435=CARTESIAN_POINT('Ctrl Pts',(-0.385003695533678,-42.3742356128,-2.31546165616534));
#73436=CARTESIAN_POINT('Ctrl Pts',(-0.368353988180329,-42.3742356128,-2.33555671215701));
#73437=CARTESIAN_POINT('Ctrl Pts',(-0.350120568954219,-42.3742356128,-2.35433014302128));
#73438=CARTESIAN_POINT('Ctrl Pts',(-0.330519834913059,-42.3742356128,-2.37155591534188));
#73439=CARTESIAN_POINT('Ctrl Pts',(-0.310822118521399,-42.3742356128,-2.3888669189546));
#73440=CARTESIAN_POINT('Ctrl Pts',(-0.289743807545843,-42.3742356128,-2.40461471280278));
#73441=CARTESIAN_POINT('Ctrl Pts',(-0.267539519104164,-42.3742356128,-2.41860932865736));
#73442=CARTESIAN_POINT('Ctrl Pts',(-0.244990950343904,-42.3742356128,-2.43282093281208));
#73443=CARTESIAN_POINT('Ctrl Pts',(-0.221281477413771,-42.3742356128,-2.44522428927903));
#73444=CARTESIAN_POINT('Ctrl Pts',(-0.196709685894568,-42.3742356128,-2.45566477541128));
#73445=CARTESIAN_POINT('Ctrl Pts',(-0.172360603756016,-42.3742356128,-2.46601063294478));
#73446=CARTESIAN_POINT('Ctrl Pts',(-0.14716515001463,-42.3742356128,-2.47442895047424));
#73447=CARTESIAN_POINT('Ctrl Pts',(-0.121439934607891,-42.3742356128,-2.48081496692291));
#73448=CARTESIAN_POINT('Ctrl Pts',(-0.0953617748833097,-42.3742356128,-2.48728859811779));
#73449=CARTESIAN_POINT('Ctrl Pts',(-0.0687395329780045,-42.3742356128,-2.49167351118973));
#73450=CARTESIAN_POINT('Ctrl Pts',(-0.0419247854849334,-42.3742356128,-2.49391070858224));
#73451=CARTESIAN_POINT('Ctrl Pts',(-0.0151100379918623,-42.3742356128,-2.49614790597475));
#73452=CARTESIAN_POINT('Ctrl Pts',(0.0118968385201095,-42.3742356128,-2.4962372385907));
#73453=CARTESIAN_POINT('Ctrl Pts',(0.0387279584952791,-42.3742356128,-2.49417248854828));
#73454=CARTESIAN_POINT('Ctrl Pts',(0.0651866464420061,-42.3742356128,-2.4921363984741));
#73455=CARTESIAN_POINT('Ctrl Pts',(0.0914718021070565,-42.3742356128,-2.48800590743246));
#73456=CARTESIAN_POINT('Ctrl Pts',(0.117243785997238,-42.3742356128,-2.4818389652788));
#73457=CARTESIAN_POINT('Ctrl Pts',(0.143035952064683,-42.3742356128,-2.47566719376003));
#73458=CARTESIAN_POINT('Ctrl Pts',(0.168313814172657,-42.3742356128,-2.46745595774278));
#73459=CARTESIAN_POINT('Ctrl Pts',(0.192758820941668,-42.3742356128,-2.45731088970016));
#73460=CARTESIAN_POINT('Ctrl Pts',(0.217190759828193,-42.3742356128,-2.44717124503739));
#73461=CARTESIAN_POINT('Ctrl Pts',(0.2407904171663,-42.3742356128,-2.43510003092528));
#73462=CARTESIAN_POINT('Ctrl Pts',(0.263266435042778,-42.3742356128,-2.42124737424211));
#73463=CARTESIAN_POINT('Ctrl Pts',(0.28569519560683,-42.3742356128,-2.40742384368477));
#73464=CARTESIAN_POINT('Ctrl Pts',(0.30700473924559,-42.3742356128,-2.39182656556059));
#73465=CARTESIAN_POINT('Ctrl Pts',(0.326936706536049,-42.3742356128,-2.37464614284886));
#73466=CARTESIAN_POINT('Ctrl Pts',(0.346909828510513,-42.3742356128,-2.35743024672612));
#73467=CARTESIAN_POINT('Ctrl Pts',(0.365499366722612,-42.3742356128,-2.33862485253807));
#73468=CARTESIAN_POINT('Ctrl Pts',(0.382481299280299,-42.3742356128,-2.31846040320672));
#73469=CARTESIAN_POINT('Ctrl Pts',(0.399249784105912,-42.3742356128,-2.29854940300218));
#73470=CARTESIAN_POINT('Ctrl Pts',(0.414450625550339,-42.3742356128,-2.27731357042829));
#73471=CARTESIAN_POINT('Ctrl Pts',(0.427906795226446,-42.3742356128,-2.25500882472017));
#73472=CARTESIAN_POINT('Ctrl Pts',(0.441619892310991,-42.3742356128,-2.23227819998046));
#73473=CARTESIAN_POINT('Ctrl Pts',(0.453520636330002,-42.3742356128,-2.2084375657962));
#73474=CARTESIAN_POINT('Ctrl Pts',(0.463467024799772,-42.3742356128,-2.18379071638894));
#73475=CARTESIAN_POINT('Ctrl Pts',(0.473413413269542,-42.3742356128,-2.15914386698167));
#73476=CARTESIAN_POINT('Ctrl Pts',(0.481405173011034,-42.3742356128,-2.13369102719235));
#73477=CARTESIAN_POINT('Ctrl Pts',(0.487350272685,-42.3742356128,-2.10776590852));
#73478=CARTESIAN_POINT('Ctrl Pts',(-0.48735027394,-40.6742356128,-2.10776590718));
#73479=CARTESIAN_POINT('Ctrl Pts',(-0.48735027394,-42.7142356128,-2.10776590718));
#73480=CARTESIAN_POINT('Ctrl Pts',(-0.427207937888,-40.6742356128,-2.37003391761));
#73481=CARTESIAN_POINT('Ctrl Pts',(-0.427207937888,-42.7142356128,-2.37003391761));
#73482=CARTESIAN_POINT('Ctrl Pts',(-0.191539291907,-40.6742356128,-2.59726293898));
#73483=CARTESIAN_POINT('Ctrl Pts',(-0.191539291907,-42.7142356128,-2.59726293898));
#73484=CARTESIAN_POINT('Ctrl Pts',(0.191539291907,-40.6742356128,-2.59726293898));
#73485=CARTESIAN_POINT('Ctrl Pts',(0.191539291907,-42.7142356128,-2.59726293898));
#73486=CARTESIAN_POINT('Ctrl Pts',(0.427207937888,-40.6742356128,-2.37003391761));
#73487=CARTESIAN_POINT('Ctrl Pts',(0.427207937888,-42.7142356128,-2.37003391761));
#73488=CARTESIAN_POINT('Ctrl Pts',(0.48735027394,-40.6742356128,-2.10776590718));
#73489=CARTESIAN_POINT('Ctrl Pts',(0.48735027394,-42.7142356128,-2.10776590718));
#73490=CARTESIAN_POINT('',(0.48735027394,-41.6742356128,-2.10776590718));
#73491=CARTESIAN_POINT('Ctrl Pts',(0.779760438305,-42.6742356128,-2.17482033117));
#73492=CARTESIAN_POINT('Ctrl Pts',(0.687897075884,-42.6742356128,-2.15375456259));
#73493=CARTESIAN_POINT('Ctrl Pts',(0.596033713464,-42.6372245963,-2.13268879401));
#73494=CARTESIAN_POINT('Ctrl Pts',(0.523424932005,-42.5627311721,-2.11603841516));
#73495=CARTESIAN_POINT('Ctrl Pts',(0.48735027394,-42.4684833924,-2.10776590718));
#73496=CARTESIAN_POINT('Ctrl Pts',(0.48735027394,-42.3742356128,-2.10776590718));
#73497=CARTESIAN_POINT('Ctrl Pts',(0.942351637347,-42.6742356128,-1.46579449204));
#73498=CARTESIAN_POINT('Ctrl Pts',(0.852970215394,-42.6742356128,-1.43390550589));
#73499=CARTESIAN_POINT('Ctrl Pts',(0.763588793442,-42.6372245963,-1.40201651973));
#73500=CARTESIAN_POINT('Ctrl Pts',(0.692941737192,-42.5627311721,-1.37681147207));
#73501=CARTESIAN_POINT('Ctrl Pts',(0.65784173486,-42.4684833924,-1.36428869651));
#73502=CARTESIAN_POINT('Ctrl Pts',(0.65784173486,-42.3742356128,-1.36428869651));
#73503=CARTESIAN_POINT('Ctrl Pts',(1.20950872503,-42.6742356128,-0.780080242745));
#73504=CARTESIAN_POINT('Ctrl Pts',(1.12418018063,-42.6742356128,-0.737834047536));
#73505=CARTESIAN_POINT('Ctrl Pts',(1.03885163623,-42.6372245963,-0.695587852327));
#73506=CARTESIAN_POINT('Ctrl Pts',(0.971407973461,-42.5627311721,-0.662196468967));
#73507=CARTESIAN_POINT('Ctrl Pts',(0.937899532468,-42.4684833924,-0.645606426859));
#73508=CARTESIAN_POINT('Ctrl Pts',(0.937899532468,-42.3742356128,-0.645606426859));
#73509=CARTESIAN_POINT('Ctrl Pts',(1.57510282168,-42.6742356128,-0.139371230964));
#73510=CARTESIAN_POINT('Ctrl Pts',(1.49532714866,-42.6742356128,-0.0873758096127));
#73511=CARTESIAN_POINT('Ctrl Pts',(1.41555147563,-42.6372245963,-0.0353803882614));
#73512=CARTESIAN_POINT('Ctrl Pts',(1.35249677314,-42.5627311721,0.00571677273303));
#73513=CARTESIAN_POINT('Ctrl Pts',(1.32116896768,-42.4684833924,0.0261353355601));
#73514=CARTESIAN_POINT('Ctrl Pts',(1.32116896768,-42.3742356128,0.0261353355601));
#73515=CARTESIAN_POINT('Ctrl Pts',(2.38346297254,-42.6742356128,0.88854638374));
#73516=CARTESIAN_POINT('Ctrl Pts',(2.31597494511,-42.6742356128,0.956184742789));
#73517=CARTESIAN_POINT('Ctrl Pts',(2.24848691768,-42.6372245963,1.02382310184));
#73518=CARTESIAN_POINT('Ctrl Pts',(2.19514441746,-42.5627311721,1.07728445262));
#73519=CARTESIAN_POINT('Ctrl Pts',(2.16864190924,-42.4684833924,1.10384596745));
#73520=CARTESIAN_POINT('Ctrl Pts',(2.16864190924,-42.3742356128,1.10384596745));
#73521=CARTESIAN_POINT('Ctrl Pts',(3.42445237435,-42.6742356128,1.67147929445));
#73522=CARTESIAN_POINT('Ctrl Pts',(3.37281026135,-42.6742356128,1.75102585468));
#73523=CARTESIAN_POINT('Ctrl Pts',(3.32116814834,-42.6372245963,1.8305724149));
#73524=CARTESIAN_POINT('Ctrl Pts',(3.28035021661,-42.5627311721,1.89344599346));
#73525=CARTESIAN_POINT('Ctrl Pts',(3.26007042322,-42.4684833924,1.92468385976));
#73526=CARTESIAN_POINT('Ctrl Pts',(3.26007042322,-42.3742356128,1.92468385976));
#73527=CARTESIAN_POINT('Ctrl Pts',(3.91792270746,-42.6742356128,1.96068148776));
#73528=CARTESIAN_POINT('Ctrl Pts',(3.87373062544,-42.6742356128,2.0445976674));
#73529=CARTESIAN_POINT('Ctrl Pts',(3.82953854342,-42.6372245963,2.12851384703));
#73530=CARTESIAN_POINT('Ctrl Pts',(3.79460919954,-42.5627311721,2.19484119775));
#73531=CARTESIAN_POINT('Ctrl Pts',(3.77725494148,-42.4684833924,2.22779498365));
#73532=CARTESIAN_POINT('Ctrl Pts',(3.77725494148,-42.3742356128,2.22779498365));
#73533=CARTESIAN_POINT('Ctrl Pts',(4.44015743262,-42.6742356128,2.19124622755));
#73534=CARTESIAN_POINT('Ctrl Pts',(4.40392272888,-42.6742356128,2.27867735624));
#73535=CARTESIAN_POINT('Ctrl Pts',(4.36768802515,-42.6372245963,2.36610848493));
#73536=CARTESIAN_POINT('Ctrl Pts',(4.33904807794,-42.5627311721,2.43521401597));
#73537=CARTESIAN_POINT('Ctrl Pts',(4.3248187884,-42.4684833924,2.46954815377));
#73538=CARTESIAN_POINT('Ctrl Pts',(4.3248187884,-42.3742356128,2.46954815377));
#73539=CARTESIAN_POINT('Ctrl Pts',(4.98144914733,-42.6742356128,2.3596116021));
#73540=CARTESIAN_POINT('Ctrl Pts',(4.95345683619,-42.6742356128,2.44960646023));
#73541=CARTESIAN_POINT('Ctrl Pts',(4.92546452504,-42.6372245963,2.53960131836));
#73542=CARTESIAN_POINT('Ctrl Pts',(4.90333940847,-42.5627311721,2.61073323444));
#73543=CARTESIAN_POINT('Ctrl Pts',(4.89234685358,-42.4684833924,2.64607413258));
#73544=CARTESIAN_POINT('Ctrl Pts',(4.89234685358,-42.3742356128,2.64607413258));
#73545=CARTESIAN_POINT('Ctrl Pts',(0.48735027394,-42.3742356128,-2.10776590718));
#73546=CARTESIAN_POINT('Ctrl Pts',(0.790651846747,-42.3742356128,-0.785131881257001));
#73547=CARTESIAN_POINT('Ctrl Pts',(1.44114622406,-42.3742356128,0.46094601538));
#73548=CARTESIAN_POINT('Ctrl Pts',(2.40362850687,-42.3742356128,1.49964984368));
#73549=CARTESIAN_POINT('Ctrl Pts',(3.59661572838,-42.3742356128,2.2430437828));
#73550=CARTESIAN_POINT('Ctrl Pts',(4.89234685393,-42.3742356128,2.64607413014));
#73551=CARTESIAN_POINT('Ctrl Pts',(0.48735027394,-40.6742356128,-2.10776590718));
#73552=CARTESIAN_POINT('Ctrl Pts',(0.48735027394,-42.7142356128,-2.10776590718));
#73553=CARTESIAN_POINT('Ctrl Pts',(0.790651846747,-40.6742356128,-0.785131881257));
#73554=CARTESIAN_POINT('Ctrl Pts',(0.790651846747,-42.7142356128,-0.785131881257));
#73555=CARTESIAN_POINT('Ctrl Pts',(1.44114622406,-40.6742356128,0.46094601538));
#73556=CARTESIAN_POINT('Ctrl Pts',(1.44114622406,-42.7142356128,0.46094601538));
#73557=CARTESIAN_POINT('Ctrl Pts',(2.40362850687,-40.6742356128,1.49964984368));
#73558=CARTESIAN_POINT('Ctrl Pts',(2.40362850687,-42.7142356128,1.49964984368));
#73559=CARTESIAN_POINT('Ctrl Pts',(3.59661572838,-40.6742356128,2.2430437828));
#73560=CARTESIAN_POINT('Ctrl Pts',(3.59661572838,-42.7142356128,2.2430437828));
#73561=CARTESIAN_POINT('Ctrl Pts',(4.89234685393,-40.6742356128,2.64607413014));
#73562=CARTESIAN_POINT('Ctrl Pts',(4.89234685393,-42.7142356128,2.64607413014));
#73563=CARTESIAN_POINT('Ctrl Pts',(6.74948971107,-42.3742356128,2.9389736393));
#73564=CARTESIAN_POINT('Ctrl Pts',(6.74948971107,-42.4684833924,2.9389736393));
#73565=CARTESIAN_POINT('Ctrl Pts',(6.74990773128,-42.5627311721,2.90196498354));
#73566=CARTESIAN_POINT('Ctrl Pts',(6.75074909582,-42.6372245963,2.82747631079));
#73567=CARTESIAN_POINT('Ctrl Pts',(6.75181357554,-42.6742356128,2.73323454275));
#73568=CARTESIAN_POINT('Ctrl Pts',(6.75287805526,-42.6742356128,2.63899277471));
#73569=CARTESIAN_POINT('Ctrl Pts',(6.66016121042,-42.3742356128,2.93796465593));
#73570=CARTESIAN_POINT('Ctrl Pts',(6.66016121042,-42.4684833924,2.93796465593));
#73571=CARTESIAN_POINT('Ctrl Pts',(6.65383637296,-42.5627311721,2.90087983603));
#73572=CARTESIAN_POINT('Ctrl Pts',(6.64110613629,-42.6372245963,2.82623787152));
#73573=CARTESIAN_POINT('Ctrl Pts',(6.62500006538,-42.6742356128,2.73180215865));
#73574=CARTESIAN_POINT('Ctrl Pts',(6.60889399448,-42.6742356128,2.63736644579));
#73575=CARTESIAN_POINT('Ctrl Pts',(6.56930976652,-42.3742356128,2.95731325003));
#73576=CARTESIAN_POINT('Ctrl Pts',(6.56930978704,-42.4684833931,2.95731325253));
#73577=CARTESIAN_POINT('Ctrl Pts',(6.55645224693,-42.5627311733,2.92167994217));
#73578=CARTESIAN_POINT('Ctrl Pts',(6.53057339717,-42.6372245978,2.8499594543));
#73579=CARTESIAN_POINT('Ctrl Pts',(6.49783190936,-42.6742356138,2.75921995253));
#73580=CARTESIAN_POINT('Ctrl Pts',(6.46509041354,-42.6742356128,2.66848045015));
#73581=CARTESIAN_POINT('Ctrl Pts',(6.48517929362,-42.3742356128,2.99677643843));
#73582=CARTESIAN_POINT('Ctrl Pts',(6.48517930736,-42.4684833932,2.99677642435));
#73583=CARTESIAN_POINT('Ctrl Pts',(6.46607746743,-42.5627311736,2.96400514186));
#73584=CARTESIAN_POINT('Ctrl Pts',(6.42763047779,-42.6372245982,2.89804241892));
#73585=CARTESIAN_POINT('Ctrl Pts',(6.37898801081,-42.6742356141,2.81458871105));
#73586=CARTESIAN_POINT('Ctrl Pts',(6.330345539,-42.6742356128,2.73113500859));
#73587=CARTESIAN_POINT('Ctrl Pts',(6.35806155931,-42.3742356128,3.0966048171));
#73588=CARTESIAN_POINT('Ctrl Pts',(6.35806154885,-42.4684833919,3.09660482782));
#73589=CARTESIAN_POINT('Ctrl Pts',(6.32947675772,-42.5627311709,3.07128279651));
#73590=CARTESIAN_POINT('Ctrl Pts',(6.27194313738,-42.6372245949,3.02031830205));
#73591=CARTESIAN_POINT('Ctrl Pts',(6.19915260335,-42.6742356119,2.95583802709));
#73592=CARTESIAN_POINT('Ctrl Pts',(6.12636207301,-42.6742356128,2.89135774799));
#73593=CARTESIAN_POINT('Ctrl Pts',(6.27916935631,-42.3742356128,3.23622606791));
#73594=CARTESIAN_POINT('Ctrl Pts',(6.27916936428,-42.4684833929,3.23622605975));
#73595=CARTESIAN_POINT('Ctrl Pts',(6.24474924576,-42.562731173,3.22125677195));
#73596=CARTESIAN_POINT('Ctrl Pts',(6.17547057799,-42.6372245974,3.19112597217));
#73597=CARTESIAN_POINT('Ctrl Pts',(6.08782042473,-42.6742356135,3.15300567784));
#73598=CARTESIAN_POINT('Ctrl Pts',(6.00017026865,-42.6742356128,3.11488538668));
#73599=CARTESIAN_POINT('Ctrl Pts',(6.25564469688,-42.3742356128,3.30224048175));
#73600=CARTESIAN_POINT('Ctrl Pts',(6.25564469441,-42.4684833903,3.30224046041));
#73601=CARTESIAN_POINT('Ctrl Pts',(6.21952273597,-42.5627311677,3.29207824683));
#73602=CARTESIAN_POINT('Ctrl Pts',(6.14681880931,-42.6372245911,3.2716308039));
#73603=CARTESIAN_POINT('Ctrl Pts',(6.05483504826,-42.6742356094,3.24575838595));
#73604=CARTESIAN_POINT('Ctrl Pts',(5.96285128692,-42.6742356128,3.21988597629));
#73605=CARTESIAN_POINT('Ctrl Pts',(6.24384239412,-42.3742356128,3.37085211609));
#73606=CARTESIAN_POINT('Ctrl Pts',(6.24384239414,-42.4684833933,3.37085211656));
#73607=CARTESIAN_POINT('Ctrl Pts',(6.20683138795,-42.5627311738,3.36573100796));
#73608=CARTESIAN_POINT('Ctrl Pts',(6.13233794388,-42.6372245985,3.35541931075));
#73609=CARTESIAN_POINT('Ctrl Pts',(6.03809015669,-42.6742356142,3.3423749178));
#73610=CARTESIAN_POINT('Ctrl Pts',(5.94384237,-42.6742356128,3.32933052468));
#73611=CARTESIAN_POINT('Ctrl Pts',(6.24384247119,-42.3742356128,3.43894174635));
#73612=CARTESIAN_POINT('Ctrl Pts',(6.24384247119,-42.4684833925,3.43894174639));
#73613=CARTESIAN_POINT('Ctrl Pts',(6.206831455,-42.5627311721,3.43894191067));
#73614=CARTESIAN_POINT('Ctrl Pts',(6.13233803133,-42.6372245964,3.43894224126));
#73615=CARTESIAN_POINT('Ctrl Pts',(6.03809025252,-42.6742356129,3.4389426595));
#73616=CARTESIAN_POINT('Ctrl Pts',(5.94384247373,-42.6742356128,3.43894307771));
#73617=CARTESIAN_POINT('',(6.74948971103925,-42.3742356128,2.93897363980053));
#73618=CARTESIAN_POINT('Origin',(6.75285456584568,-42.3763569074475,2.64111394033772));
#73619=CARTESIAN_POINT('',(6.24384247076,-42.3742356128,3.43894174696));
#73620=CARTESIAN_POINT('Ctrl Pts',(6.74948971107,-42.3742356128,2.9389736393));
#73621=CARTESIAN_POINT('Ctrl Pts',(6.59129069763,-42.3742356128,2.93718674963));
#73622=CARTESIAN_POINT('Ctrl Pts',(6.43081292755,-42.3742356128,2.99918925876));
#73623=CARTESIAN_POINT('Ctrl Pts',(6.30765353814,-42.3742356128,3.12096539428));
#73624=CARTESIAN_POINT('Ctrl Pts',(6.24384247076,-42.3742356128,3.28073264221));
#73625=CARTESIAN_POINT('Ctrl Pts',(6.24384247076,-42.3742356128,3.43894174696));
#73626=CARTESIAN_POINT('Origin',(5.94596381538561,-42.3763569542133,3.43894399659967));
#73627=CARTESIAN_POINT('Ctrl Pts',(6.24384247076,-40.6742356128,3.43894174696));
#73628=CARTESIAN_POINT('Ctrl Pts',(6.24384247076,-42.7142356128,3.43894174696));
#73629=CARTESIAN_POINT('Ctrl Pts',(6.24384247076,-40.6742356128,3.28073264221));
#73630=CARTESIAN_POINT('Ctrl Pts',(6.24384247076,-42.7142356128,3.28073264221));
#73631=CARTESIAN_POINT('Ctrl Pts',(6.30765353814,-40.6742356128,3.12096539428));
#73632=CARTESIAN_POINT('Ctrl Pts',(6.30765353814,-42.7142356128,3.12096539428));
#73633=CARTESIAN_POINT('Ctrl Pts',(6.43081292755,-40.6742356128,2.99918925876));
#73634=CARTESIAN_POINT('Ctrl Pts',(6.43081292755,-42.7142356128,2.99918925876));
#73635=CARTESIAN_POINT('Ctrl Pts',(6.59129069763,-40.6742356128,2.93718674963));
#73636=CARTESIAN_POINT('Ctrl Pts',(6.59129069763,-42.7142356128,2.93718674963));
#73637=CARTESIAN_POINT('Ctrl Pts',(6.74948971107,-40.6742356128,2.9389736393));
#73638=CARTESIAN_POINT('Ctrl Pts',(6.74948971107,-42.7142356128,2.9389736393));
#73639=CARTESIAN_POINT('',(6.74948971107,-41.6742356128,2.9389736393));
#73640=CARTESIAN_POINT('',(6.24384247076,-41.5242356128,3.43894174696));
#73641=CARTESIAN_POINT('Ctrl Pts',(0.487165434784,-42.3742356128,-5.01265134236));
#73642=CARTESIAN_POINT('Ctrl Pts',(0.487165434783,-42.4684833925,-5.01265134236));
#73643=CARTESIAN_POINT('Ctrl Pts',(0.523241153367,-42.5627311721,-5.00438346023));
#73644=CARTESIAN_POINT('Ctrl Pts',(0.595852069376,-42.6372245964,-4.98774239199));
#73645=CARTESIAN_POINT('Ctrl Pts',(0.687718132381,-42.6742356129,-4.96668840305));
#73646=CARTESIAN_POINT('Ctrl Pts',(0.779584195372,-42.6742356128,-4.94563441411));
#73647=CARTESIAN_POINT('Ctrl Pts',(0.81460270388,-42.3742356128,-6.44137631405));
#73648=CARTESIAN_POINT('Ctrl Pts',(0.814602703711,-42.4684833979,-6.44137631333));
#73649=CARTESIAN_POINT('Ctrl Pts',(0.848817867564,-42.562731183,-6.4249900945));
#73650=CARTESIAN_POINT('Ctrl Pts',(0.917683903123,-42.6372246092,-6.39200862181));
#73651=CARTESIAN_POINT('Ctrl Pts',(1.0048120379,-42.6742356214,-6.35028117911));
#73652=CARTESIAN_POINT('Ctrl Pts',(1.09194016947,-42.6742356128,-6.30855373743));
#73653=CARTESIAN_POINT('Ctrl Pts',(1.54487166721,-42.3742356128,-7.77811177525));
#73654=CARTESIAN_POINT('Ctrl Pts',(1.5448713568,-42.4684833875,-7.77811123165));
#73655=CARTESIAN_POINT('Ctrl Pts',(1.57490766806,-42.5627311622,-7.75405190508));
#73656=CARTESIAN_POINT('Ctrl Pts',(1.6353633393,-42.6372245846,-7.70562798343));
#73657=CARTESIAN_POINT('Ctrl Pts',(1.71185094269,-42.6742356051,-7.64436300383));
#73658=CARTESIAN_POINT('Ctrl Pts',(1.7883386711,-42.6742356128,-7.58309823758));
#73659=CARTESIAN_POINT('Ctrl Pts',(2.64459800142,-42.3742356128,-8.86954551869));
#73660=CARTESIAN_POINT('Ctrl Pts',(2.64459795101,-42.468483394,-8.86954558844));
#73661=CARTESIAN_POINT('Ctrl Pts',(2.66838977506,-42.5627311752,-8.83932950434));
#73662=CARTESIAN_POINT('Ctrl Pts',(2.7162764821,-42.6372246,-8.7785122786));
#73663=CARTESIAN_POINT('Ctrl Pts',(2.77686194922,-42.6742356153,-8.70156739678));
#73664=CARTESIAN_POINT('Ctrl Pts',(2.83744743521,-42.6742356128,-8.62462248786));
#73665=CARTESIAN_POINT('Ctrl Pts',(5.32102214868,-42.3742356128,-10.3065086991));
#73666=CARTESIAN_POINT('Ctrl Pts',(5.32102219883,-42.4684833909,-10.3065086297));
#73667=CARTESIAN_POINT('Ctrl Pts',(5.32957386707,-42.562731169,-10.2680846534));
#73668=CARTESIAN_POINT('Ctrl Pts',(5.34678608834,-42.6372245927,-10.1907475223));
#73669=CARTESIAN_POINT('Ctrl Pts',(5.36856264868,-42.6742356104,-10.0929019242));
#73670=CARTESIAN_POINT('Ctrl Pts',(5.39033919025,-42.6742356128,-9.99505635309));
#73671=CARTESIAN_POINT('Ctrl Pts',(8.35327745821,-42.3742356128,-10.1381955831));
#73672=CARTESIAN_POINT('Ctrl Pts',(8.35327740833,-42.468483394,-10.1381956522));
#73673=CARTESIAN_POINT('Ctrl Pts',(8.34456301547,-42.5627311751,-10.1007555191));
#73674=CARTESIAN_POINT('Ctrl Pts',(8.32702327197,-42.6372246,-10.0253981883));
#73675=CARTESIAN_POINT('Ctrl Pts',(8.30483233612,-42.6742356153,-9.93005741943));
#73676=CARTESIAN_POINT('Ctrl Pts',(8.28264141894,-42.6742356128,-9.83471662374));
#73677=CARTESIAN_POINT('Ctrl Pts',(9.80390850636,-42.3742356128,-9.62023799647));
#73678=CARTESIAN_POINT('Ctrl Pts',(9.8039083944,-42.4684833936,-9.62023813852));
#73679=CARTESIAN_POINT('Ctrl Pts',(9.78693869153,-42.5627311743,-9.58574518127));
#73680=CARTESIAN_POINT('Ctrl Pts',(9.7527832879,-42.637224599,-9.51631977282));
#73681=CARTESIAN_POINT('Ctrl Pts',(9.70957053609,-42.6742356146,-9.42848387231));
#73682=CARTESIAN_POINT('Ctrl Pts',(9.66635782899,-42.6742356128,-9.34064791616));
#73683=CARTESIAN_POINT('Ctrl Pts',(12.2505485061,-42.3742356128,-7.83535708458));
#73684=CARTESIAN_POINT('Ctrl Pts',(12.250548618,-42.4684833913,-7.83535694254));
#73685=CARTESIAN_POINT('Ctrl Pts',(12.2196394502,-42.5627311698,-7.81100596215));
#73686=CARTESIAN_POINT('Ctrl Pts',(12.1574273028,-42.6372245937,-7.76199402851));
#73687=CARTESIAN_POINT('Ctrl Pts',(12.0787175117,-42.6742356111,-7.69998507205));
#73688=CARTESIAN_POINT('Ctrl Pts',(12.0000076759,-42.6742356128,-7.63797617123));
#73689=CARTESIAN_POINT('Ctrl Pts',(13.4125693644,-42.3742356128,-5.03814078999));
#73690=CARTESIAN_POINT('Ctrl Pts',(13.4125692525,-42.4684833936,-5.03814093202));
#73691=CARTESIAN_POINT('Ctrl Pts',(13.3750518255,-42.5627311743,-5.02973844738));
#73692=CARTESIAN_POINT('Ctrl Pts',(13.2995392669,-42.637224599,-5.01282628628));
#73693=CARTESIAN_POINT('Ctrl Pts',(13.204002165,-42.6742356146,-4.99142922913));
#73694=CARTESIAN_POINT('Ctrl Pts',(13.1084651078,-42.6742356128,-4.97003211634));
#73695=CARTESIAN_POINT('Ctrl Pts',(13.5759583006,-42.3742356128,-3.50667079674));
#73696=CARTESIAN_POINT('Ctrl Pts',(13.5759583811,-42.4684833893,-3.50667095934));
#73697=CARTESIAN_POINT('Ctrl Pts',(13.5375192988,-42.5627311657,-3.50696861096));
#73698=CARTESIAN_POINT('Ctrl Pts',(13.4601513294,-42.6372245889,-3.50756750816));
#73699=CARTESIAN_POINT('Ctrl Pts',(13.3622667292,-42.6742356079,-3.50832512382));
#73700=CARTESIAN_POINT('Ctrl Pts',(13.2643820967,-42.6742356128,-3.50908267685));
#73701=CARTESIAN_POINT('Ctrl Pts',(13.0288342859,-42.3742356128,-0.519322029858));
#73702=CARTESIAN_POINT('Ctrl Pts',(13.028834205,-42.4684833956,-0.519321866398));
#73703=CARTESIAN_POINT('Ctrl Pts',(12.9934845041,-42.5627311784,-0.536648062284));
#73704=CARTESIAN_POINT('Ctrl Pts',(12.9223350964,-42.6372246039,-0.571521327091));
#73705=CARTESIAN_POINT('Ctrl Pts',(12.8323181043,-42.6742356178,-0.6156424721));
#73706=CARTESIAN_POINT('Ctrl Pts',(12.7423011448,-42.6742356128,-0.659763680066));
#73707=CARTESIAN_POINT('Ctrl Pts',(11.004586804,-42.3742356128,1.74562563294));
#73708=CARTESIAN_POINT('Ctrl Pts',(11.0045868854,-42.4684833892,1.74562546861));
#73709=CARTESIAN_POINT('Ctrl Pts',(10.9807897791,-42.5627311657,1.71542042139));
#73710=CARTESIAN_POINT('Ctrl Pts',(10.9328922473,-42.6372245888,1.65462581836));
#73711=CARTESIAN_POINT('Ctrl Pts',(10.8722931303,-42.6742356078,1.57770964821));
#73712=CARTESIAN_POINT('Ctrl Pts',(10.8116939805,-42.6742356128,1.50079354136));
#73713=CARTESIAN_POINT('Ctrl Pts',(9.68588827029,-42.3742356128,2.55889041883));
#73714=CARTESIAN_POINT('Ctrl Pts',(9.6858884488,-42.4684834004,2.55889048283));
#73715=CARTESIAN_POINT('Ctrl Pts',(9.66954131867,-42.5627311879,2.52404881238));
#73716=CARTESIAN_POINT('Ctrl Pts',(9.63663914597,-42.637224615,2.45392163988));
#73717=CARTESIAN_POINT('Ctrl Pts',(9.5950115686,-42.6742356253,2.36519792666));
#73718=CARTESIAN_POINT('Ctrl Pts',(9.55338392126,-42.6742356128,2.27647419301));
#73719=CARTESIAN_POINT('Ctrl Pts',(8.21519030725,-42.3742356128,2.95553030618));
#73720=CARTESIAN_POINT('Ctrl Pts',(8.21519030799,-42.468483387,2.95553030619));
#73721=CARTESIAN_POINT('Ctrl Pts',(8.20727993006,-42.5627311611,2.91842756273));
#73722=CARTESIAN_POINT('Ctrl Pts',(8.19135808192,-42.6372245834,2.84374951081));
#73723=CARTESIAN_POINT('Ctrl Pts',(8.17121418034,-42.6742356043,2.7492681436));
#73724=CARTESIAN_POINT('Ctrl Pts',(8.15107027851,-42.6742356128,2.65478677305));
#73725=CARTESIAN_POINT('Ctrl Pts',(6.74948971076,-42.3742356128,2.9389736413));
#73726=CARTESIAN_POINT('Ctrl Pts',(6.74948971076,-42.4684833924,2.9389736413));
#73727=CARTESIAN_POINT('Ctrl Pts',(6.74990776683,-42.562731172,2.90196498592));
#73728=CARTESIAN_POINT('Ctrl Pts',(6.75074920355,-42.6372245963,2.82747631396));
#73729=CARTESIAN_POINT('Ctrl Pts',(6.75181377459,-42.6742356128,2.7332345469));
#73730=CARTESIAN_POINT('Ctrl Pts',(6.75287834563,-42.6742356128,2.63899277983));
#73731=CARTESIAN_POINT('',(0.487165436324921,-42.3742356128,-5.01265134230888));
#73732=CARTESIAN_POINT('Origin',(0.777516257206663,-42.3763569108251,-4.9461071823497));
#73733=CARTESIAN_POINT('Ctrl Pts',(0.4871654368,-42.3742356128,-5.0126513422));
#73734=CARTESIAN_POINT('Ctrl Pts',(0.813757598474,-42.3742356128,-6.43768308726));
#73735=CARTESIAN_POINT('Ctrl Pts',(1.54099672242,-42.3742356128,-7.77089360944));
#73736=CARTESIAN_POINT('Ctrl Pts',(2.63582398808,-42.3742356128,-8.86093046307));
#73737=CARTESIAN_POINT('Ctrl Pts',(5.30859738244,-42.3742356128,-10.303702289));
#73738=CARTESIAN_POINT('Ctrl Pts',(8.3416246802,-42.3742356128,-10.1422911046));
#73739=CARTESIAN_POINT('Ctrl Pts',(9.79740146658,-42.3742356128,-9.62504741726));
#73740=CARTESIAN_POINT('Ctrl Pts',(12.2523240225,-42.3742356128,-7.83656666427));
#73741=CARTESIAN_POINT('Ctrl Pts',(13.4155860878,-42.3742356128,-5.03083511496));
#73742=CARTESIAN_POINT('Ctrl Pts',(13.5772083053,-42.3742356128,-3.49437641304));
#73743=CARTESIAN_POINT('Ctrl Pts',(13.0232255151,-42.3742356128,-0.50800550047));
#73744=CARTESIAN_POINT('Ctrl Pts',(10.9941845663,-42.3742356128,1.75214958001));
#73745=CARTESIAN_POINT('Ctrl Pts',(9.67790042305,-42.3742356128,2.56099019349));
#73746=CARTESIAN_POINT('Ctrl Pts',(8.21137385808,-42.3742356128,2.95548591471));
#73747=CARTESIAN_POINT('Ctrl Pts',(6.74948971107,-42.3742356128,2.9389736393));
#73748=CARTESIAN_POINT('Ctrl Pts',(6.74948971107,-40.6742356128,2.9389736393));
#73749=CARTESIAN_POINT('Ctrl Pts',(6.74948971107,-42.7142356128,2.9389736393));
#73750=CARTESIAN_POINT('Ctrl Pts',(8.21137385808,-40.6742356128,2.95548591471));
#73751=CARTESIAN_POINT('Ctrl Pts',(8.21137385808,-42.7142356128,2.95548591471));
#73752=CARTESIAN_POINT('Ctrl Pts',(9.67790042305,-40.6742356128,2.56099019349));
#73753=CARTESIAN_POINT('Ctrl Pts',(9.67790042305,-42.7142356128,2.56099019349));
#73754=CARTESIAN_POINT('Ctrl Pts',(10.9941845663,-40.6742356128,1.75214958001));
#73755=CARTESIAN_POINT('Ctrl Pts',(10.9941845663,-42.7142356128,1.75214958001));
#73756=CARTESIAN_POINT('Ctrl Pts',(13.0232255151,-40.6742356128,-0.50800550047));
#73757=CARTESIAN_POINT('Ctrl Pts',(13.0232255151,-42.7142356128,-0.50800550047));
#73758=CARTESIAN_POINT('Ctrl Pts',(13.5772083053,-40.6742356128,-3.49437641304));
#73759=CARTESIAN_POINT('Ctrl Pts',(13.5772083053,-42.7142356128,-3.49437641304));
#73760=CARTESIAN_POINT('Ctrl Pts',(13.4155860878,-40.6742356128,-5.03083511496));
#73761=CARTESIAN_POINT('Ctrl Pts',(13.4155860878,-42.7142356128,-5.03083511496));
#73762=CARTESIAN_POINT('Ctrl Pts',(12.2523240225,-40.6742356128,-7.83656666427));
#73763=CARTESIAN_POINT('Ctrl Pts',(12.2523240225,-42.7142356128,-7.83656666427));
#73764=CARTESIAN_POINT('Ctrl Pts',(9.79740146658,-40.6742356128,-9.62504741726));
#73765=CARTESIAN_POINT('Ctrl Pts',(9.79740146658,-42.7142356128,-9.62504741726));
#73766=CARTESIAN_POINT('Ctrl Pts',(8.3416246802,-40.6742356128,-10.1422911046));
#73767=CARTESIAN_POINT('Ctrl Pts',(8.3416246802,-42.7142356128,-10.1422911046));
#73768=CARTESIAN_POINT('Ctrl Pts',(5.30859738244,-40.6742356128,-10.303702289));
#73769=CARTESIAN_POINT('Ctrl Pts',(5.30859738244,-42.7142356128,-10.303702289));
#73770=CARTESIAN_POINT('Ctrl Pts',(2.63582398808,-40.6742356128,-8.86093046307));
#73771=CARTESIAN_POINT('Ctrl Pts',(2.63582398808,-42.7142356128,-8.86093046307));
#73772=CARTESIAN_POINT('Ctrl Pts',(1.54099672242,-40.6742356128,-7.77089360944));
#73773=CARTESIAN_POINT('Ctrl Pts',(1.54099672242,-42.7142356128,-7.77089360944));
#73774=CARTESIAN_POINT('Ctrl Pts',(0.813757598474,-40.6742356128,-6.43768308726));
#73775=CARTESIAN_POINT('Ctrl Pts',(0.813757598474,-42.7142356128,-6.43768308726));
#73776=CARTESIAN_POINT('Ctrl Pts',(0.4871654368,-40.6742356128,-5.0126513422));
#73777=CARTESIAN_POINT('Ctrl Pts',(0.4871654368,-42.7142356128,-5.0126513422));
#73778=CARTESIAN_POINT('',(0.4871654368,-41.6742356128,-5.0126513422));
#73779=CARTESIAN_POINT('Ctrl Pts',(-6.10622663544E-16,-42.3742356128,-4.62434669465));
#73780=CARTESIAN_POINT('Ctrl Pts',(-5.82867087928E-16,-42.4684833924,-4.62434669465));
#73781=CARTESIAN_POINT('Ctrl Pts',(-1.33226762955E-15,-42.5627311721,-4.58733567815));
#73782=CARTESIAN_POINT('Ctrl Pts',(-2.69229083472E-15,-42.6372245963,-4.51284225387));
#73783=CARTESIAN_POINT('Ctrl Pts',(-4.55191440096E-15,-42.6742356128,-4.41859447426));
#73784=CARTESIAN_POINT('Ctrl Pts',(-6.27276008913E-15,-42.6742356128,-4.32434669465));
#73785=CARTESIAN_POINT('Ctrl Pts',(0.0757509451836,-42.3742356128,-4.62434669465));
#73786=CARTESIAN_POINT('Ctrl Pts',(0.0757509451836,-42.4684833924,-4.62434669465));
#73787=CARTESIAN_POINT('Ctrl Pts',(0.0814347989626,-42.5627311721,-4.58733567684));
#73788=CARTESIAN_POINT('Ctrl Pts',(0.0928749048103,-42.6372245963,-4.51284225387));
#73789=CARTESIAN_POINT('Ctrl Pts',(0.107348724535,-42.6742356128,-4.41859447426));
#73790=CARTESIAN_POINT('Ctrl Pts',(0.121822544253,-42.6742356128,-4.32434669465));
#73791=CARTESIAN_POINT('Ctrl Pts',(0.152161902464,-42.3742356128,-4.63889679318));
#73792=CARTESIAN_POINT('Ctrl Pts',(0.152161789276,-42.4684833943,-4.63889677644));
#73793=CARTESIAN_POINT('Ctrl Pts',(0.163415494185,-42.5627311758,-4.60297257201));
#73794=CARTESIAN_POINT('Ctrl Pts',(0.186066359196,-42.6372246007,-4.53066662124));
#73795=CARTESIAN_POINT('Ctrl Pts',(0.214723913443,-42.6742356158,-4.43918641142));
#73796=CARTESIAN_POINT('Ctrl Pts',(0.243381511931,-42.6742356128,-4.34770620929));
#73797=CARTESIAN_POINT('Ctrl Pts',(0.224510888247,-42.3742356128,-4.66787112912));
#73798=CARTESIAN_POINT('Ctrl Pts',(0.224510927626,-42.4684833926,-4.66787117042));
#73799=CARTESIAN_POINT('Ctrl Pts',(0.241126667402,-42.5627311724,-4.63407065981));
#73800=CARTESIAN_POINT('Ctrl Pts',(0.27456862703,-42.6372245967,-4.56603424662));
#73801=CARTESIAN_POINT('Ctrl Pts',(0.316879247465,-42.6742356131,-4.47995777227));
#73802=CARTESIAN_POINT('Ctrl Pts',(0.359189852064,-42.6742356128,-4.39388128157));
#73803=CARTESIAN_POINT('Ctrl Pts',(0.339412867472,-42.3742356128,-4.74197790598));
#73804=CARTESIAN_POINT('Ctrl Pts',(0.3394128372,-42.4684833923,-4.74197787423));
#73805=CARTESIAN_POINT('Ctrl Pts',(0.364563818788,-42.5627311718,-4.71367989972));
#73806=CARTESIAN_POINT('Ctrl Pts',(0.415186981668,-42.637224596,-4.656727276));
#73807=CARTESIAN_POINT('Ctrl Pts',(0.479234194727,-42.6742356126,-4.58467027499));
#73808=CARTESIAN_POINT('Ctrl Pts',(0.543281419947,-42.6742356128,-4.51261328653));
#73809=CARTESIAN_POINT('Ctrl Pts',(0.423242092027,-42.3742356128,-4.84894453188));
#73810=CARTESIAN_POINT('Ctrl Pts',(0.423242115298,-42.4684833925,-4.84894455629));
#73811=CARTESIAN_POINT('Ctrl Pts',(0.454600156263,-42.5627311722,-4.82857509388));
#73812=CARTESIAN_POINT('Ctrl Pts',(0.517714979555,-42.6372245966,-4.78757386924));
#73813=CARTESIAN_POINT('Ctrl Pts',(0.597566998874,-42.674235613,-4.73570101093));
#73814=CARTESIAN_POINT('Ctrl Pts',(0.677419008856,-42.6742356128,-4.68382814298));
#73815=CARTESIAN_POINT('Ctrl Pts',(0.452677771562,-42.3742356128,-4.90062212276));
#73816=CARTESIAN_POINT('Ctrl Pts',(0.452677723796,-42.4684833907,-4.90062199961));
#73817=CARTESIAN_POINT('Ctrl Pts',(0.486189267495,-42.5627311685,-4.88403912837));
#73818=CARTESIAN_POINT('Ctrl Pts',(0.553641781761,-42.6372245921,-4.85067372199));
#73819=CARTESIAN_POINT('Ctrl Pts',(0.638980484601,-42.6742356101,-4.80845568264));
#73820=CARTESIAN_POINT('Ctrl Pts',(0.724319207107,-42.6742356128,-4.76623769098));
#73821=CARTESIAN_POINT('Ctrl Pts',(0.474132994671,-42.3742356128,-4.95578655666));
#73822=CARTESIAN_POINT('Ctrl Pts',(0.474132994712,-42.468483392,-4.95578655679));
#73823=CARTESIAN_POINT('Ctrl Pts',(0.509236440803,-42.5627311712,-4.94327645524));
#73824=CARTESIAN_POINT('Ctrl Pts',(0.579888733321,-42.6372245954,-4.91808932499));
#73825=CARTESIAN_POINT('Ctrl Pts',(0.66927749198,-42.6742356122,-4.88622619544));
#73826=CARTESIAN_POINT('Ctrl Pts',(0.75866625092,-42.6742356128,-4.85436306591));
#73827=CARTESIAN_POINT('Ctrl Pts',(0.487165436864,-42.3742356128,-5.01265134225));
#73828=CARTESIAN_POINT('Ctrl Pts',(0.487165436863,-42.4684833925,-5.01265134225));
#73829=CARTESIAN_POINT('Ctrl Pts',(0.52324113624,-42.5627311721,-5.00438337628));
#73830=CARTESIAN_POINT('Ctrl Pts',(0.595852013591,-42.6372245963,-4.98774213931));
#73831=CARTESIAN_POINT('Ctrl Pts',(0.687718027696,-42.6742356128,-4.96668793687));
#73832=CARTESIAN_POINT('Ctrl Pts',(0.779584041801,-42.6742356128,-4.94563373444));
#73833=CARTESIAN_POINT('',(-6.66133814775E-16,-42.3742356128,-4.62434669465));
#73834=CARTESIAN_POINT('Origin',(-6.2003040155756E-7,-42.3763569029672,
-4.32646798455307));
#73835=CARTESIAN_POINT('Ctrl Pts',(-6.66133814775E-16,-42.3742356128,-4.62434669465));
#73836=CARTESIAN_POINT('Ctrl Pts',(0.134351406801,-42.3742356128,-4.62434669465));
#73837=CARTESIAN_POINT('Ctrl Pts',(0.269654391195,-42.3742356128,-4.67008903963));
#73838=CARTESIAN_POINT('Ctrl Pts',(0.38229629568,-42.3742356128,-4.75983578098));
#73839=CARTESIAN_POINT('Ctrl Pts',(0.457108114206,-42.3742356128,-4.88150110685));
#73840=CARTESIAN_POINT('Ctrl Pts',(0.4871654368,-42.3742356128,-5.0126513422));
#73841=CARTESIAN_POINT('Ctrl Pts',(0.4871654368,-40.6742356128,-5.0126513422));
#73842=CARTESIAN_POINT('Ctrl Pts',(0.4871654368,-42.7142356128,-5.0126513422));
#73843=CARTESIAN_POINT('Ctrl Pts',(0.457108114206,-40.6742356128,-4.88150110685));
#73844=CARTESIAN_POINT('Ctrl Pts',(0.457108114206,-42.7142356128,-4.88150110685));
#73845=CARTESIAN_POINT('Ctrl Pts',(0.38229629568,-40.6742356128,-4.75983578098));
#73846=CARTESIAN_POINT('Ctrl Pts',(0.38229629568,-42.7142356128,-4.75983578098));
#73847=CARTESIAN_POINT('Ctrl Pts',(0.269654391195,-40.6742356128,-4.67008903963));
#73848=CARTESIAN_POINT('Ctrl Pts',(0.269654391195,-42.7142356128,-4.67008903963));
#73849=CARTESIAN_POINT('Ctrl Pts',(0.134351406801,-40.6742356128,-4.62434669465));
#73850=CARTESIAN_POINT('Ctrl Pts',(0.134351406801,-42.7142356128,-4.62434669465));
#73851=CARTESIAN_POINT('Ctrl Pts',(-1.11022302463E-15,-40.6742356128,-4.62434669465));
#73852=CARTESIAN_POINT('Ctrl Pts',(-1.11022302463E-15,-42.7142356128,-4.62434669465));
#73853=CARTESIAN_POINT('',(-6.66133814775E-16,-41.6742356128,-4.62434669465));
#73854=CARTESIAN_POINT('Ctrl Pts',(-0.4871654368,-42.3742356128,-5.0126513422));
#73855=CARTESIAN_POINT('Ctrl Pts',(-0.4871654368,-42.4684833924,-5.0126513422));
#73856=CARTESIAN_POINT('Ctrl Pts',(-0.523241147327,-42.5627311721,-5.00438342513));
#73857=CARTESIAN_POINT('Ctrl Pts',(-0.595852047118,-42.6372245963,-4.98774228657));
#73858=CARTESIAN_POINT('Ctrl Pts',(-0.687718089613,-42.6742356128,-4.96668820865));
#73859=CARTESIAN_POINT('Ctrl Pts',(-0.779584132109,-42.6742356128,-4.94563413072));
#73860=CARTESIAN_POINT('Ctrl Pts',(-0.470219247563,-42.3742356128,-4.93870940343));
#73861=CARTESIAN_POINT('Ctrl Pts',(-0.470219247563,-42.4684833924,-4.93870940343));
#73862=CARTESIAN_POINT('Ctrl Pts',(-0.5050271879,-42.5627311721,-4.92490977213));
#73863=CARTESIAN_POINT('Ctrl Pts',(-0.575086395474,-42.6372245963,-4.89713474521));
#73864=CARTESIAN_POINT('Ctrl Pts',(-0.663724083576,-42.6742356128,-4.86199426829));
#73865=CARTESIAN_POINT('Ctrl Pts',(-0.752361771679,-42.6742356128,-4.82685379139));
#73866=CARTESIAN_POINT('Ctrl Pts',(-0.438960828789,-42.3742356128,-4.86744285923));
#73867=CARTESIAN_POINT('Ctrl Pts',(-0.438960870115,-42.4684833944,-4.86744296509));
#73868=CARTESIAN_POINT('Ctrl Pts',(-0.471468366068,-42.562731176,-4.84845573386));
#73869=CARTESIAN_POINT('Ctrl Pts',(-0.536897355711,-42.6372246009,-4.81023932414));
#73870=CARTESIAN_POINT('Ctrl Pts',(-0.619676938308,-42.6742356159,-4.76188852036));
#73871=CARTESIAN_POINT('Ctrl Pts',(-0.70245650358,-42.6742356128,-4.71353767549));
#73872=CARTESIAN_POINT('Ctrl Pts',(-0.394558742266,-42.3742356128,-4.80337215755));
#73873=CARTESIAN_POINT('Ctrl Pts',(-0.394558692852,-42.4684833926,-4.80337212861));
#73874=CARTESIAN_POINT('Ctrl Pts',(-0.42379715787,-42.5627311723,-4.77962978503));
#73875=CARTESIAN_POINT('Ctrl Pts',(-0.482651660681,-42.6372245967,-4.73184272758));
#73876=CARTESIAN_POINT('Ctrl Pts',(-0.557111231681,-42.6742356131,-4.67138339935));
#73877=CARTESIAN_POINT('Ctrl Pts',(-0.631570822294,-42.6742356128,-4.61092408283));
#73878=CARTESIAN_POINT('Ctrl Pts',(-0.296664664887,-42.3742356128,-4.70791349655));
#73879=CARTESIAN_POINT('Ctrl Pts',(-0.296664702856,-42.4684833923,-4.70791351879));
#73880=CARTESIAN_POINT('Ctrl Pts',(-0.318633564797,-42.5627311718,-4.67707994976));
#73881=CARTESIAN_POINT('Ctrl Pts',(-0.362847138464,-42.6372245961,-4.61502009393));
#73882=CARTESIAN_POINT('Ctrl Pts',(-0.418786998681,-42.6742356127,-4.53650302527));
#73883=CARTESIAN_POINT('Ctrl Pts',(-0.474726843846,-42.6742356128,-4.45798594764));
#73884=CARTESIAN_POINT('Ctrl Pts',(-0.173690010613,-42.3742356128,-4.6500860894));
#73885=CARTESIAN_POINT('Ctrl Pts',(-0.173689981439,-42.4684833925,-4.65008607231));
#73886=CARTESIAN_POINT('Ctrl Pts',(-0.186545459408,-42.5627311722,-4.61497252538));
#73887=CARTESIAN_POINT('Ctrl Pts',(-0.212423173742,-42.6372245965,-4.54429820168));
#73888=CARTESIAN_POINT('Ctrl Pts',(-0.245161968871,-42.674235613,-4.45488230314));
#73889=CARTESIAN_POINT('Ctrl Pts',(-0.277900775553,-42.6742356128,-4.36546641149));
#73890=CARTESIAN_POINT('Ctrl Pts',(-0.116772148725,-42.3742356128,-4.63293650019));
#73891=CARTESIAN_POINT('Ctrl Pts',(-0.11677228042,-42.4684833908,-4.63293651935));
#73892=CARTESIAN_POINT('Ctrl Pts',(-0.125457169651,-42.5627311687,-4.59656929085));
#73893=CARTESIAN_POINT('Ctrl Pts',(-0.14292537866,-42.6372245923,-4.52337168016));
#73894=CARTESIAN_POINT('Ctrl Pts',(-0.165030820729,-42.6742356102,-4.43076330315));
#73895=CARTESIAN_POINT('Ctrl Pts',(-0.187136211538,-42.6742356128,-4.33815491762));
#73896=CARTESIAN_POINT('Ctrl Pts',(-0.0582513837293,-42.3742356128,-4.62434672797));
#73897=CARTESIAN_POINT('Ctrl Pts',(-0.0582513835551,-42.4684833921,-4.62434672797));
#73898=CARTESIAN_POINT('Ctrl Pts',(-0.0626101237973,-42.5627311713,-4.58733574114));
#73899=CARTESIAN_POINT('Ctrl Pts',(-0.0713911309205,-42.6372245954,-4.51284233288));
#73900=CARTESIAN_POINT('Ctrl Pts',(-0.0824973438866,-42.6742356122,-4.4185945918));
#73901=CARTESIAN_POINT('Ctrl Pts',(-0.0936035567729,-42.6742356128,-4.32434685045));
#73902=CARTESIAN_POINT('Ctrl Pts',(7.0763099266E-11,-42.3742356128,-4.6243466946));
#73903=CARTESIAN_POINT('Ctrl Pts',(6.59831173003E-11,-42.4684833925,-4.6243466946));
#73904=CARTESIAN_POINT('Ctrl Pts',(-4.72553275957E-8,-42.5627311721,-4.58733567804));
#73905=CARTESIAN_POINT('Ctrl Pts',(-1.42494814745E-7,-42.6372245963,-4.51284225365));
#73906=CARTESIAN_POINT('Ctrl Pts',(-2.62987247912E-7,-42.6742356128,-4.4185944739));
#73907=CARTESIAN_POINT('Ctrl Pts',(-3.8347780408E-7,-42.6742356128,-4.32434669416));
#73908=CARTESIAN_POINT('',(-0.4871654368,-42.3742356128,-5.0126513422));
#73909=CARTESIAN_POINT('Origin',(-0.777515787161492,-42.3763569160989,-4.94610519328655));
#73910=CARTESIAN_POINT('Ctrl Pts',(-0.4871654368,-42.3742356128,-5.0126513422));
#73911=CARTESIAN_POINT('Ctrl Pts',(-0.457108114206,-42.3742356128,-4.88150110685));
#73912=CARTESIAN_POINT('Ctrl Pts',(-0.38229629568,-42.3742356128,-4.75983578098));
#73913=CARTESIAN_POINT('Ctrl Pts',(-0.269654391195,-42.3742356128,-4.67008903963));
#73914=CARTESIAN_POINT('Ctrl Pts',(-0.134351406801,-42.3742356128,-4.62434669465));
#73915=CARTESIAN_POINT('Ctrl Pts',(-6.66133814775E-16,-42.3742356128,-4.62434669465));
#73916=CARTESIAN_POINT('Ctrl Pts',(-6.17561557448E-16,-40.6742356128,-4.62434669465));
#73917=CARTESIAN_POINT('Ctrl Pts',(-6.17561557448E-16,-42.7142356128,-4.62434669465));
#73918=CARTESIAN_POINT('Ctrl Pts',(-0.134351406801,-40.6742356128,-4.62434669465));
#73919=CARTESIAN_POINT('Ctrl Pts',(-0.134351406801,-42.7142356128,-4.62434669465));
#73920=CARTESIAN_POINT('Ctrl Pts',(-0.269654391195,-40.6742356128,-4.67008903963));
#73921=CARTESIAN_POINT('Ctrl Pts',(-0.269654391195,-42.7142356128,-4.67008903963));
#73922=CARTESIAN_POINT('Ctrl Pts',(-0.38229629568,-40.6742356128,-4.75983578098));
#73923=CARTESIAN_POINT('Ctrl Pts',(-0.38229629568,-42.7142356128,-4.75983578098));
#73924=CARTESIAN_POINT('Ctrl Pts',(-0.457108114206,-40.6742356128,-4.88150110685));
#73925=CARTESIAN_POINT('Ctrl Pts',(-0.457108114206,-42.7142356128,-4.88150110685));
#73926=CARTESIAN_POINT('Ctrl Pts',(-0.4871654368,-40.6742356128,-5.0126513422));
#73927=CARTESIAN_POINT('Ctrl Pts',(-0.4871654368,-42.7142356128,-5.0126513422));
#73928=CARTESIAN_POINT('',(-0.4871654368,-41.6742356128,-5.0126513422));
#73929=CARTESIAN_POINT('Ctrl Pts',(-6.74948971107,-42.3742356128,2.9389736393));
#73930=CARTESIAN_POINT('Ctrl Pts',(-6.74948971107,-42.4684833924,2.9389736393));
#73931=CARTESIAN_POINT('Ctrl Pts',(-6.74990773128,-42.5627311721,2.90196498354));
#73932=CARTESIAN_POINT('Ctrl Pts',(-6.75074909582,-42.6372245963,2.82747631079));
#73933=CARTESIAN_POINT('Ctrl Pts',(-6.75181357554,-42.6742356128,2.73323454275));
#73934=CARTESIAN_POINT('Ctrl Pts',(-6.75287805526,-42.6742356128,2.63899277471));
#73935=CARTESIAN_POINT('Ctrl Pts',(-8.20750926282,-42.3742356128,2.95544226333));
#73936=CARTESIAN_POINT('Ctrl Pts',(-8.20750926282,-42.4684833924,2.95544226333));
#73937=CARTESIAN_POINT('Ctrl Pts',(-8.19962531608,-42.5627311721,2.91833983518));
#73938=CARTESIAN_POINT('Ctrl Pts',(-8.18375700837,-42.6372245963,2.84366242333));
#73939=CARTESIAN_POINT('Ctrl Pts',(-8.16368070265,-42.6742356128,2.74918186586));
#73940=CARTESIAN_POINT('Ctrl Pts',(-8.14360439693,-42.6742356128,2.6547013084));
#73941=CARTESIAN_POINT('Ctrl Pts',(-9.67024722863,-42.3742356128,2.5630230066));
#73942=CARTESIAN_POINT('Ctrl Pts',(-9.67024704898,-42.4684833943,2.56302294195));
#73943=CARTESIAN_POINT('Ctrl Pts',(-9.65401144272,-42.5627311758,2.52816442735));
#73944=CARTESIAN_POINT('Ctrl Pts',(-9.62133366522,-42.6372246008,2.45800350109));
#73945=CARTESIAN_POINT('Ctrl Pts',(-9.579990421,-42.6742356158,2.36923716228));
#73946=CARTESIAN_POINT('Ctrl Pts',(-9.53864724787,-42.6742356128,2.28047084985));
#73947=CARTESIAN_POINT('Ctrl Pts',(-10.9836939618,-42.3742356128,1.75867662573));
#73948=CARTESIAN_POINT('Ctrl Pts',(-10.9836938807,-42.4684833913,1.75867678874));
#73949=CARTESIAN_POINT('Ctrl Pts',(-10.9600136456,-42.5627311698,1.72838802594));
#73950=CARTESIAN_POINT('Ctrl Pts',(-10.912351671,-42.6372245937,1.66742452742));
#73951=CARTESIAN_POINT('Ctrl Pts',(-10.852050622,-42.6742356111,1.59029447444));
#73952=CARTESIAN_POINT('Ctrl Pts',(-10.7917496044,-42.6742356128,1.51316435682));
#73953=CARTESIAN_POINT('Ctrl Pts',(-13.0127891544,-42.3742356128,-0.491277894672));
#73954=CARTESIAN_POINT('Ctrl Pts',(-13.0127892356,-42.4684833936,-0.491278057762));
#73955=CARTESIAN_POINT('Ctrl Pts',(-12.9775329168,-42.5627311743,-0.508754582936));
#73956=CARTESIAN_POINT('Ctrl Pts',(-12.9065711376,-42.637224599,-0.543930023858));
#73957=CARTESIAN_POINT('Ctrl Pts',(-12.8167914846,-42.6742356146,-0.588433278065));
#73958=CARTESIAN_POINT('Ctrl Pts',(-12.7270118002,-42.6742356128,-0.632936467611));
#73959=CARTESIAN_POINT('Ctrl Pts',(-13.5757021091,-42.3742356128,-3.4678350886));
#73960=CARTESIAN_POINT('Ctrl Pts',(-13.5757020279,-42.4684833913,-3.46783492542));
#73961=CARTESIAN_POINT('Ctrl Pts',(-13.5372624578,-42.5627311698,-3.46836301962));
#73962=CARTESIAN_POINT('Ctrl Pts',(-13.4598938305,-42.6372245937,-3.46942613318));
#73963=CARTESIAN_POINT('Ctrl Pts',(-13.3620084433,-42.6742356111,-3.47077126553));
#73964=CARTESIAN_POINT('Ctrl Pts',(-13.2641230876,-42.6742356128,-3.47211646258));
#73965=CARTESIAN_POINT('Ctrl Pts',(-13.4210719777,-42.3742356128,-5.00117407132));
#73966=CARTESIAN_POINT('Ctrl Pts',(-13.4210720895,-42.4684833921,-5.00117392804));
#73967=CARTESIAN_POINT('Ctrl Pts',(-13.383504567,-42.5627311713,-4.99297868135));
#73968=CARTESIAN_POINT('Ctrl Pts',(-13.3078909057,-42.6372245955,-4.97648398449));
#73969=CARTESIAN_POINT('Ctrl Pts',(-13.2122257538,-42.6742356123,-4.95561526881));
#73970=CARTESIAN_POINT('Ctrl Pts',(-13.1165605577,-42.6742356128,-4.93474660917));
#73971=CARTESIAN_POINT('Ctrl Pts',(-12.2737890543,-42.3742356128,-7.80629649793));
#73972=CARTESIAN_POINT('Ctrl Pts',(-12.2737889425,-42.4684833928,-7.80629664121));
#73973=CARTESIAN_POINT('Ctrl Pts',(-12.2427485647,-42.5627311728,-7.78211510142));
#73974=CARTESIAN_POINT('Ctrl Pts',(-12.1802726,-42.6372245972,-7.73344385831));
#73975=CARTESIAN_POINT('Ctrl Pts',(-12.1012291684,-42.6742356134,-7.67186576452));
#73976=CARTESIAN_POINT('Ctrl Pts',(-12.022185781,-42.6742356128,-7.61028761468));
#73977=CARTESIAN_POINT('Ctrl Pts',(-9.83534450901,-42.3742356128,-9.60498420728));
#73978=CARTESIAN_POINT('Ctrl Pts',(-9.83534462085,-42.4684833921,-9.604984064));
#73979=CARTESIAN_POINT('Ctrl Pts',(-9.8181953458,-42.5627311713,-9.57057329056));
#73980=CARTESIAN_POINT('Ctrl Pts',(-9.7836782372,-42.6372245955,-9.50131364513));
#73981=CARTESIAN_POINT('Ctrl Pts',(-9.74000772596,-42.6742356123,-9.4136876382));
#73982=CARTESIAN_POINT('Ctrl Pts',(-9.69633717052,-42.6742356128,-9.3260616873));
#73983=CARTESIAN_POINT('Ctrl Pts',(-8.38661907184,-42.3742356128,-10.1306138711));
#73984=CARTESIAN_POINT('Ctrl Pts',(-8.38661911955,-42.4684833948,-10.1306137972));
#73985=CARTESIAN_POINT('Ctrl Pts',(-8.37771609534,-42.5627311767,-10.0932252432));
#73986=CARTESIAN_POINT('Ctrl Pts',(-8.35979658423,-42.6372246018,-10.017971977));
#73987=CARTESIAN_POINT('Ctrl Pts',(-8.33712510637,-42.6742356165,-9.92276292417));
#73988=CARTESIAN_POINT('Ctrl Pts',(-8.3144536084,-42.6742356128,-9.82755390065));
#73989=CARTESIAN_POINT('Ctrl Pts',(-5.34778827807,-42.3742356128,-10.3144544476));
#73990=CARTESIAN_POINT('Ctrl Pts',(-5.34778822992,-42.4684833901,-10.3144545222));
#73991=CARTESIAN_POINT('Ctrl Pts',(-5.35618547139,-42.5627311674,-10.2759765996));
#73992=CARTESIAN_POINT('Ctrl Pts',(-5.37308697531,-42.6372245908,-10.198530638));
#73993=CARTESIAN_POINT('Ctrl Pts',(-5.39447048864,-42.6742356092,-10.1005472936));
#73994=CARTESIAN_POINT('Ctrl Pts',(-5.41585402228,-42.6742356128,-10.0025639196));
#73995=CARTESIAN_POINT('Ctrl Pts',(-2.6588016357,-42.3742356128,-8.88354817531));
#73996=CARTESIAN_POINT('Ctrl Pts',(-2.65880168429,-42.4684833948,-8.88354810004));
#73997=CARTESIAN_POINT('Ctrl Pts',(-2.68251543773,-42.5627311768,-8.85326127917));
#73998=CARTESIAN_POINT('Ctrl Pts',(-2.73024490553,-42.6372246019,-8.79230193136));
#73999=CARTESIAN_POINT('Ctrl Pts',(-2.79063136862,-42.6742356165,-8.71517729568));
#74000=CARTESIAN_POINT('Ctrl Pts',(-2.85101781122,-42.6742356128,-8.63805268983));
#74001=CARTESIAN_POINT('Ctrl Pts',(-1.5511450484,-42.3742356128,-7.78971751005));
#74002=CARTESIAN_POINT('Ctrl Pts',(-1.55114537045,-42.4684833818,-7.78971807464));
#74003=CARTESIAN_POINT('Ctrl Pts',(-1.58113889708,-42.5627311508,-7.76555835799));
#74004=CARTESIAN_POINT('Ctrl Pts',(-1.64150761259,-42.6372245712,-7.71693072276));
#74005=CARTESIAN_POINT('Ctrl Pts',(-1.71788484767,-42.6742355961,-7.65540746012));
#74006=CARTESIAN_POINT('Ctrl Pts',(-1.79426196246,-42.6742356128,-7.59388397371));
#74007=CARTESIAN_POINT('Ctrl Pts',(-0.815993189233,-42.3742356128,-6.44741976998));
#74008=CARTESIAN_POINT('Ctrl Pts',(-0.815993188532,-42.4684833972,-6.44741976695));
#74009=CARTESIAN_POINT('Ctrl Pts',(-0.850205838116,-42.5627311816,-6.43102299012));
#74010=CARTESIAN_POINT('Ctrl Pts',(-0.919066859411,-42.6372246076,-6.39802046996));
#74011=CARTESIAN_POINT('Ctrl Pts',(-1.00618863168,-42.6742356204,-6.35626631563));
#74012=CARTESIAN_POINT('Ctrl Pts',(-1.09331040135,-42.6742356128,-6.31451216314));
#74013=CARTESIAN_POINT('Ctrl Pts',(-0.48716542938,-42.3742356128,-5.01265134292));
#74014=CARTESIAN_POINT('Ctrl Pts',(-0.487165429388,-42.4684833924,-5.01265134296));
#74015=CARTESIAN_POINT('Ctrl Pts',(-0.523241090791,-42.562731172,-5.00438321101));
#74016=CARTESIAN_POINT('Ctrl Pts',(-0.595851891697,-42.6372245963,-4.9877416399));
#74017=CARTESIAN_POINT('Ctrl Pts',(-0.687717809092,-42.6742356128,-4.9666870147));
#74018=CARTESIAN_POINT('Ctrl Pts',(-0.779583726501,-42.6742356128,-4.94563238948));
#74019=CARTESIAN_POINT('',(-6.74948971107,-42.3742356128,2.9389736393));
#74020=CARTESIAN_POINT('Origin',(-6.75285593709817,-42.3763569039433,2.641113951342));
#74021=CARTESIAN_POINT('Ctrl Pts',(-6.74948971107,-42.3742356128,2.9389736393));
#74022=CARTESIAN_POINT('Ctrl Pts',(-8.21137385808,-42.3742356128,2.95548591471));
#74023=CARTESIAN_POINT('Ctrl Pts',(-9.67790042305,-42.3742356128,2.56099019349));
#74024=CARTESIAN_POINT('Ctrl Pts',(-10.9941845663,-42.3742356128,1.75214958001));
#74025=CARTESIAN_POINT('Ctrl Pts',(-13.0232255151,-42.3742356128,-0.50800550047));
#74026=CARTESIAN_POINT('Ctrl Pts',(-13.5772083053,-42.3742356128,-3.49437641304));
#74027=CARTESIAN_POINT('Ctrl Pts',(-13.4155860878,-42.3742356128,-5.03083511496));
#74028=CARTESIAN_POINT('Ctrl Pts',(-12.2523240225,-42.3742356128,-7.83656666427));
#74029=CARTESIAN_POINT('Ctrl Pts',(-9.79740146658,-42.3742356128,-9.62504741726));
#74030=CARTESIAN_POINT('Ctrl Pts',(-8.3416246802,-42.3742356128,-10.1422911046));
#74031=CARTESIAN_POINT('Ctrl Pts',(-5.30859738244,-42.3742356128,-10.303702289));
#74032=CARTESIAN_POINT('Ctrl Pts',(-2.63582398808,-42.3742356128,-8.86093046307));
#74033=CARTESIAN_POINT('Ctrl Pts',(-1.54099672242,-42.3742356128,-7.77089360944));
#74034=CARTESIAN_POINT('Ctrl Pts',(-0.813757598474,-42.3742356128,-6.43768308726));
#74035=CARTESIAN_POINT('Ctrl Pts',(-0.4871654368,-42.3742356128,-5.0126513422));
#74036=CARTESIAN_POINT('Ctrl Pts',(-0.4871654368,-40.6742356128,-5.0126513422));
#74037=CARTESIAN_POINT('Ctrl Pts',(-0.4871654368,-42.7142356128,-5.0126513422));
#74038=CARTESIAN_POINT('Ctrl Pts',(-0.813757598474,-40.6742356128,-6.43768308726));
#74039=CARTESIAN_POINT('Ctrl Pts',(-0.813757598474,-42.7142356128,-6.43768308726));
#74040=CARTESIAN_POINT('Ctrl Pts',(-1.54099672242,-40.6742356128,-7.77089360944));
#74041=CARTESIAN_POINT('Ctrl Pts',(-1.54099672242,-42.7142356128,-7.77089360944));
#74042=CARTESIAN_POINT('Ctrl Pts',(-2.63582398808,-40.6742356128,-8.86093046307));
#74043=CARTESIAN_POINT('Ctrl Pts',(-2.63582398808,-42.7142356128,-8.86093046307));
#74044=CARTESIAN_POINT('Ctrl Pts',(-5.30859738244,-40.6742356128,-10.303702289));
#74045=CARTESIAN_POINT('Ctrl Pts',(-5.30859738244,-42.7142356128,-10.303702289));
#74046=CARTESIAN_POINT('Ctrl Pts',(-8.3416246802,-40.6742356128,-10.1422911046));
#74047=CARTESIAN_POINT('Ctrl Pts',(-8.3416246802,-42.7142356128,-10.1422911046));
#74048=CARTESIAN_POINT('Ctrl Pts',(-9.79740146658,-40.6742356128,-9.62504741726));
#74049=CARTESIAN_POINT('Ctrl Pts',(-9.79740146658,-42.7142356128,-9.62504741726));
#74050=CARTESIAN_POINT('Ctrl Pts',(-12.2523240225,-40.6742356128,-7.83656666427));
#74051=CARTESIAN_POINT('Ctrl Pts',(-12.2523240225,-42.7142356128,-7.83656666427));
#74052=CARTESIAN_POINT('Ctrl Pts',(-13.4155860878,-40.6742356128,-5.03083511496));
#74053=CARTESIAN_POINT('Ctrl Pts',(-13.4155860878,-42.7142356128,-5.03083511496));
#74054=CARTESIAN_POINT('Ctrl Pts',(-13.5772083053,-40.6742356128,-3.49437641304));
#74055=CARTESIAN_POINT('Ctrl Pts',(-13.5772083053,-42.7142356128,-3.49437641304));
#74056=CARTESIAN_POINT('Ctrl Pts',(-13.0232255151,-40.6742356128,-0.50800550047));
#74057=CARTESIAN_POINT('Ctrl Pts',(-13.0232255151,-42.7142356128,-0.50800550047));
#74058=CARTESIAN_POINT('Ctrl Pts',(-10.9941845663,-40.6742356128,1.75214958001));
#74059=CARTESIAN_POINT('Ctrl Pts',(-10.9941845663,-42.7142356128,1.75214958001));
#74060=CARTESIAN_POINT('Ctrl Pts',(-9.67790042305,-40.6742356128,2.56099019349));
#74061=CARTESIAN_POINT('Ctrl Pts',(-9.67790042305,-42.7142356128,2.56099019349));
#74062=CARTESIAN_POINT('Ctrl Pts',(-8.21137385808,-40.6742356128,2.95548591471));
#74063=CARTESIAN_POINT('Ctrl Pts',(-8.21137385808,-42.7142356128,2.95548591471));
#74064=CARTESIAN_POINT('Ctrl Pts',(-6.74948971107,-40.6742356128,2.9389736393));
#74065=CARTESIAN_POINT('Ctrl Pts',(-6.74948971107,-42.7142356128,2.9389736393));
#74066=CARTESIAN_POINT('',(-6.74948971107,-41.6742356128,2.9389736393));
#74067=CARTESIAN_POINT('Ctrl Pts',(-6.24384247076,-42.3742356128,3.43894174696));
#74068=CARTESIAN_POINT('Ctrl Pts',(-6.24384247076,-42.4684833924,3.43894174696));
#74069=CARTESIAN_POINT('Ctrl Pts',(-6.20683145426,-42.5627311721,3.43894174696));
#74070=CARTESIAN_POINT('Ctrl Pts',(-6.13233802997,-42.6372245963,3.43894174696));
#74071=CARTESIAN_POINT('Ctrl Pts',(-6.03809025037,-42.6742356128,3.43894174696));
#74072=CARTESIAN_POINT('Ctrl Pts',(-5.94384247076,-42.6742356128,3.43894174696));
#74073=CARTESIAN_POINT('Ctrl Pts',(-6.24384247076,-42.3742356128,3.34960754815));
#74074=CARTESIAN_POINT('Ctrl Pts',(-6.24384247076,-42.4684833924,3.34960754815));
#74075=CARTESIAN_POINT('Ctrl Pts',(-6.20683145206,-42.5627311721,3.34286426034));
#74076=CARTESIAN_POINT('Ctrl Pts',(-6.13233802997,-42.6372245963,3.32929179344));
#74077=CARTESIAN_POINT('Ctrl Pts',(-6.03809025037,-42.6742356128,3.31212014752));
#74078=CARTESIAN_POINT('Ctrl Pts',(-5.94384247076,-42.6742356128,3.29494850162));
#74079=CARTESIAN_POINT('Ctrl Pts',(-6.26421595059,-42.3742356128,3.2589804315));
#74080=CARTESIAN_POINT('Ctrl Pts',(-6.26421595287,-42.4684833931,3.25898045204));
#74081=CARTESIAN_POINT('Ctrl Pts',(-6.2287301346,-42.5627311733,3.24572127232));
#74082=CARTESIAN_POINT('Ctrl Pts',(-6.15730650956,-42.6372245978,3.21903402757));
#74083=CARTESIAN_POINT('Ctrl Pts',(-6.06694259369,-42.6742356138,3.18526977261));
#74084=CARTESIAN_POINT('Ctrl Pts',(-5.97657867728,-42.6742356128,3.15150550965));
#74085=CARTESIAN_POINT('Ctrl Pts',(-6.30462683184,-42.3742356128,3.17530104105));
#74086=CARTESIAN_POINT('Ctrl Pts',(-6.30462681761,-42.4684833932,3.17530105464));
#74087=CARTESIAN_POINT('Ctrl Pts',(-6.27207337078,-42.5627311736,3.1558302985));
#74088=CARTESIAN_POINT('Ctrl Pts',(-6.20654909404,-42.6372245982,3.11664074649));
#74089=CARTESIAN_POINT('Ctrl Pts',(-6.12365010064,-42.6742356141,3.06705881587));
#74090=CARTESIAN_POINT('Ctrl Pts',(-6.0407511127,-42.6742356128,3.01747688048));
#74091=CARTESIAN_POINT('Ctrl Pts',(-6.40588457178,-42.3742356128,3.0493189246));
#74092=CARTESIAN_POINT('Ctrl Pts',(-6.40588458262,-42.4684833919,3.04931891426));
#74093=CARTESIAN_POINT('Ctrl Pts',(-6.38088701684,-42.5627311709,3.02044994721));
#74094=CARTESIAN_POINT('Ctrl Pts',(-6.33057558549,-42.6372245949,2.96234437914));
#74095=CARTESIAN_POINT('Ctrl Pts',(-6.26692155466,-42.6742356119,2.88883021682));
#74096=CARTESIAN_POINT('Ctrl Pts',(-6.20326751965,-42.6742356128,2.81531605813));
#74097=CARTESIAN_POINT('Ctrl Pts',(-6.54638796335,-42.3742356128,2.97200870323));
#74098=CARTESIAN_POINT('Ctrl Pts',(-6.5463879551,-42.4684833929,2.97200871111));
#74099=CARTESIAN_POINT('Ctrl Pts',(-6.53180837948,-42.562731173,2.93742171773));
#74100=CARTESIAN_POINT('Ctrl Pts',(-6.50246196815,-42.6372245974,2.86780715714));
#74101=CARTESIAN_POINT('Ctrl Pts',(-6.46533406827,-42.6742356135,2.77973204569));
#74102=CARTESIAN_POINT('Ctrl Pts',(-6.42820617159,-42.6742356128,2.69165693147));
#74103=CARTESIAN_POINT('Ctrl Pts',(-6.61266386529,-42.3742356128,2.94923114283));
#74104=CARTESIAN_POINT('Ctrl Pts',(-6.61266384398,-42.4684833903,2.94923114012));
#74105=CARTESIAN_POINT('Ctrl Pts',(-6.60291025736,-42.5627311677,2.91299670879));
#74106=CARTESIAN_POINT('Ctrl Pts',(-6.58328527175,-42.6372245911,2.84006647627));
#74107=CARTESIAN_POINT('Ctrl Pts',(-6.55845341287,-42.6742356094,2.74779636686));
#74108=CARTESIAN_POINT('Ctrl Pts',(-6.53362156228,-42.6742356128,2.65552625724));
#74109=CARTESIAN_POINT('Ctrl Pts',(-6.68140442414,-42.3742356128,2.93820452565));
#74110=CARTESIAN_POINT('Ctrl Pts',(-6.68140442461,-42.4684833933,2.93820452567));
#74111=CARTESIAN_POINT('Ctrl Pts',(-6.67670166275,-42.5627311738,2.90113803996));
#74112=CARTESIAN_POINT('Ctrl Pts',(-6.66723198803,-42.6372245985,2.82653288217));
#74113=CARTESIAN_POINT('Ctrl Pts',(-6.65525290692,-42.6742356142,2.7321437769));
#74114=CARTESIAN_POINT('Ctrl Pts',(-6.64327382563,-42.6742356128,2.63775467212));
#74115=CARTESIAN_POINT('Ctrl Pts',(-6.74948971045,-42.3742356128,2.93897363973));
#74116=CARTESIAN_POINT('Ctrl Pts',(-6.7494897105,-42.4684833925,2.93897363973));
#74117=CARTESIAN_POINT('Ctrl Pts',(-6.74990789497,-42.5627311721,2.90196498613));
#74118=CARTESIAN_POINT('Ctrl Pts',(-6.75074959007,-42.6372245964,2.82747631774));
#74119=CARTESIAN_POINT('Ctrl Pts',(-6.75181448799,-42.6742356129,2.73323455521));
#74120=CARTESIAN_POINT('Ctrl Pts',(-6.7528793859,-42.6742356128,2.63899279271));
#74121=CARTESIAN_POINT('',(-6.24384247076,-42.3742356128,3.43894174696));
#74122=CARTESIAN_POINT('Origin',(-5.94596376190762,-42.3763569039501,3.43894174696));
#74123=CARTESIAN_POINT('Ctrl Pts',(-6.24384247076,-42.3742356128,3.43894174696));
#74124=CARTESIAN_POINT('Ctrl Pts',(-6.24384247076,-42.3742356128,3.28073264221));
#74125=CARTESIAN_POINT('Ctrl Pts',(-6.30765353814,-42.3742356128,3.12096539428));
#74126=CARTESIAN_POINT('Ctrl Pts',(-6.43081292755,-42.3742356128,2.99918925876));
#74127=CARTESIAN_POINT('Ctrl Pts',(-6.59129069763,-42.3742356128,2.93718674963));
#74128=CARTESIAN_POINT('Ctrl Pts',(-6.74948971107,-42.3742356128,2.9389736393));
#74129=CARTESIAN_POINT('Ctrl Pts',(-6.74948971107,-40.6742356128,2.9389736393));
#74130=CARTESIAN_POINT('Ctrl Pts',(-6.74948971107,-42.7142356128,2.9389736393));
#74131=CARTESIAN_POINT('Ctrl Pts',(-6.59129069763,-40.6742356128,2.93718674963));
#74132=CARTESIAN_POINT('Ctrl Pts',(-6.59129069763,-42.7142356128,2.93718674963));
#74133=CARTESIAN_POINT('Ctrl Pts',(-6.43081292755,-40.6742356128,2.99918925876));
#74134=CARTESIAN_POINT('Ctrl Pts',(-6.43081292755,-42.7142356128,2.99918925876));
#74135=CARTESIAN_POINT('Ctrl Pts',(-6.30765353814,-40.6742356128,3.12096539428));
#74136=CARTESIAN_POINT('Ctrl Pts',(-6.30765353814,-42.7142356128,3.12096539428));
#74137=CARTESIAN_POINT('Ctrl Pts',(-6.24384247076,-40.6742356128,3.28073264221));
#74138=CARTESIAN_POINT('Ctrl Pts',(-6.24384247076,-42.7142356128,3.28073264221));
#74139=CARTESIAN_POINT('Ctrl Pts',(-6.24384247076,-40.6742356128,3.43894174696));
#74140=CARTESIAN_POINT('Ctrl Pts',(-6.24384247076,-42.7142356128,3.43894174696));
#74141=CARTESIAN_POINT('',(-6.24384247076,-41.5242356128,3.43894174696));
#74142=CARTESIAN_POINT('Origin',(-5.94384247076,-42.3742356128,1.43032185727));
#74143=CARTESIAN_POINT('',(-6.2438424664575,-42.3742356128,6.9209196413125));
#74144=CARTESIAN_POINT('Origin',(-5.94596379715983,-42.3763569539716,6.92091847872721));
#74145=CARTESIAN_POINT('',(-6.24384247076,-42.3742356128,5.17993069345));
#74146=CARTESIAN_POINT('Origin',(-6.24384247076,-40.6742356128,3.43894174696));
#74147=CARTESIAN_POINT('',(-6.24384247076,-41.6742356128,6.92091963994));
#74148=CARTESIAN_POINT('Ctrl Pts',(-3.99680288865E-15,-42.3742356128,13.1643460036));
#74149=CARTESIAN_POINT('Ctrl Pts',(-3.99680288865E-15,-42.4684833924,13.1643460036));
#74150=CARTESIAN_POINT('Ctrl Pts',(-3.99680288865E-15,-42.5627311721,13.127334987));
#74151=CARTESIAN_POINT('Ctrl Pts',(-3.5527136788E-15,-42.6372245963,13.0528415628));
#74152=CARTESIAN_POINT('Ctrl Pts',(-2.44249065418E-15,-42.6742356128,12.9585937832));
#74153=CARTESIAN_POINT('Ctrl Pts',(-2.22044604925E-15,-42.6742356128,12.8643460036));
#74154=CARTESIAN_POINT('Ctrl Pts',(-0.830355780019,-42.3742356128,13.1643460036));
#74155=CARTESIAN_POINT('Ctrl Pts',(-0.830355780019,-42.4684833924,13.1643460036));
#74156=CARTESIAN_POINT('Ctrl Pts',(-0.825449681018,-42.5627311721,13.1273349871));
#74157=CARTESIAN_POINT('Ctrl Pts',(-0.815574996274,-42.6372245963,13.0528415628));
#74158=CARTESIAN_POINT('Ctrl Pts',(-0.803081717631,-42.6742356128,12.9585937832));
#74159=CARTESIAN_POINT('Ctrl Pts',(-0.790588438987,-42.6742356128,12.8643460036));
#74160=CARTESIAN_POINT('Ctrl Pts',(-1.66094634074,-42.3742356128,13.0267583307));
#74161=CARTESIAN_POINT('Ctrl Pts',(-1.66094608426,-42.4684833982,13.0267583306));
#74162=CARTESIAN_POINT('Ctrl Pts',(-1.65110706951,-42.5627311836,12.9905602371));
#74163=CARTESIAN_POINT('Ctrl Pts',(-1.63130403909,-42.6372246099,12.9177030127));
#74164=CARTESIAN_POINT('Ctrl Pts',(-1.60624974683,-42.6742356219,12.825525327));
#74165=CARTESIAN_POINT('Ctrl Pts',(-1.58119555591,-42.6742356128,12.7333476449));
#74166=CARTESIAN_POINT('Ctrl Pts',(-2.46049232399,-42.3742356128,12.7504708603));
#74167=CARTESIAN_POINT('Ctrl Pts',(-2.46049212731,-42.4684833922,12.7504710156));
#74168=CARTESIAN_POINT('Ctrl Pts',(-2.44590069233,-42.5627311716,12.7159220787));
#74169=CARTESIAN_POINT('Ctrl Pts',(-2.41653221863,-42.6372245958,12.6463839634));
#74170=CARTESIAN_POINT('Ctrl Pts',(-2.37937585833,-42.6742356125,12.5584054672));
#74171=CARTESIAN_POINT('Ctrl Pts',(-2.34221957571,-42.6742356128,12.4704269092));
#74172=CARTESIAN_POINT('Ctrl Pts',(-4.20512684159,-42.3742356128,11.7964487758));
#74173=CARTESIAN_POINT('Ctrl Pts',(-4.20512710956,-42.4684833928,11.7964485642));
#74174=CARTESIAN_POINT('Ctrl Pts',(-4.18019508788,-42.5627311727,11.7675458902));
#74175=CARTESIAN_POINT('Ctrl Pts',(-4.13001317043,-42.6372245971,11.7093727067));
#74176=CARTESIAN_POINT('Ctrl Pts',(-4.06652372142,-42.6742356133,11.6357731294));
#74177=CARTESIAN_POINT('Ctrl Pts',(-4.00303416657,-42.6742356128,11.5621736363));
#74178=CARTESIAN_POINT('Ctrl Pts',(-5.47475449391,-42.3742356128,10.2366927474));
#74179=CARTESIAN_POINT('Ctrl Pts',(-5.47475412882,-42.468483392,10.2366930358));
#74180=CARTESIAN_POINT('Ctrl Pts',(-5.44231202099,-42.5627311712,10.2170346303));
#74181=CARTESIAN_POINT('Ctrl Pts',(-5.37701505136,-42.6372245953,10.1774670535));
#74182=CARTESIAN_POINT('Ctrl Pts',(-5.29440268823,-42.6742356122,10.1274066844));
#74183=CARTESIAN_POINT('Ctrl Pts',(-5.21179046929,-42.6742356128,10.0773462007));
#74184=CARTESIAN_POINT('Ctrl Pts',(-5.98838818076,-42.3742356128,9.18394779498));
#74185=CARTESIAN_POINT('Ctrl Pts',(-5.98838818346,-42.4684833776,9.18394826002));
#74186=CARTESIAN_POINT('Ctrl Pts',(-5.9528871956,-42.5627311424,9.17049598399));
#74187=CARTESIAN_POINT('Ctrl Pts',(-5.88143305972,-42.6372245614,9.14341966516));
#74188=CARTESIAN_POINT('Ctrl Pts',(-5.79103052636,-42.6742355896,9.1091628388));
#74189=CARTESIAN_POINT('Ctrl Pts',(-5.70062798276,-42.6742356128,9.0749058287));
#74190=CARTESIAN_POINT('Ctrl Pts',(-6.24384251168,-42.3742356128,8.05203845412));
#74191=CARTESIAN_POINT('Ctrl Pts',(-6.24384251169,-42.4684833956,8.05203845264));
#74192=CARTESIAN_POINT('Ctrl Pts',(-6.2068314946,-42.5627311784,8.04537359323));
#74193=CARTESIAN_POINT('Ctrl Pts',(-6.13233806792,-42.6372246038,8.03195889811));
#74194=CARTESIAN_POINT('Ctrl Pts',(-6.03809028705,-42.6742356178,8.01498689923));
#74195=CARTESIAN_POINT('Ctrl Pts',(-5.94384250813,-42.6742356128,7.99801490093));
#74196=CARTESIAN_POINT('Ctrl Pts',(-6.24384245355,-42.3742356128,6.9209196436));
#74197=CARTESIAN_POINT('Ctrl Pts',(-6.24384245355,-42.4684833924,6.92091964364));
#74198=CARTESIAN_POINT('Ctrl Pts',(-6.20683143735,-42.562731172,6.92091949894));
#74199=CARTESIAN_POINT('Ctrl Pts',(-6.13233801368,-42.6372245963,6.92091920766));
#74200=CARTESIAN_POINT('Ctrl Pts',(-6.03809023484,-42.6742356128,6.92091883911));
#74201=CARTESIAN_POINT('Ctrl Pts',(-5.94384245598,-42.6742356128,6.92091847055));
#74202=CARTESIAN_POINT('',(3.5527148831751E-15,-42.3742356128,13.1643460036));
#74203=CARTESIAN_POINT('Origin',(-1.89812050115279E-6,-42.3763568746686,
12.8664672572934));
#74204=CARTESIAN_POINT('Ctrl Pts',(3.5527136788E-15,-42.3742356128,13.1643460036));
#74205=CARTESIAN_POINT('Ctrl Pts',(-1.96184634686,-42.3742356128,13.1643460036));
#74206=CARTESIAN_POINT('Ctrl Pts',(-3.92510661379,-42.3742356128,12.3963108842));
#74207=CARTESIAN_POINT('Ctrl Pts',(-5.47580735138,-42.3742356128,10.8456101466));
#74208=CARTESIAN_POINT('Ctrl Pts',(-6.24384247076,-42.3742356128,8.88234987966));
#74209=CARTESIAN_POINT('Ctrl Pts',(-6.24384247076,-42.3742356128,6.92091963994));
#74210=CARTESIAN_POINT('Ctrl Pts',(-6.24384247076,-40.6742356128,6.92091963994));
#74211=CARTESIAN_POINT('Ctrl Pts',(-6.24384247076,-42.7142356128,6.92091963994));
#74212=CARTESIAN_POINT('Ctrl Pts',(-6.24384247076,-40.6742356128,8.88234987966));
#74213=CARTESIAN_POINT('Ctrl Pts',(-6.24384247076,-42.7142356128,8.88234987966));
#74214=CARTESIAN_POINT('Ctrl Pts',(-5.47580735138,-40.6742356128,10.8456101466));
#74215=CARTESIAN_POINT('Ctrl Pts',(-5.47580735138,-42.7142356128,10.8456101466));
#74216=CARTESIAN_POINT('Ctrl Pts',(-3.92510661379,-40.6742356128,12.3963108842));
#74217=CARTESIAN_POINT('Ctrl Pts',(-3.92510661379,-42.7142356128,12.3963108842));
#74218=CARTESIAN_POINT('Ctrl Pts',(-1.96184634686,-40.6742356128,13.1643460036));
#74219=CARTESIAN_POINT('Ctrl Pts',(-1.96184634686,-42.7142356128,13.1643460036));
#74220=CARTESIAN_POINT('Ctrl Pts',(5.44009282066E-15,-40.6742356128,13.1643460036));
#74221=CARTESIAN_POINT('Ctrl Pts',(5.44009282066E-15,-42.7142356128,13.1643460036));
#74222=CARTESIAN_POINT('',(3.5527136788E-15,-41.6742356128,13.1643460036));
#74223=CARTESIAN_POINT('Ctrl Pts',(6.24384247076,-42.3742356128,6.92091963994));
#74224=CARTESIAN_POINT('Ctrl Pts',(6.24384247076,-42.4684833924,6.92091963994));
#74225=CARTESIAN_POINT('Ctrl Pts',(6.20683145426,-42.5627311721,6.92091963994));
#74226=CARTESIAN_POINT('Ctrl Pts',(6.13233802997,-42.6372245963,6.92091963994));
#74227=CARTESIAN_POINT('Ctrl Pts',(6.03809025037,-42.6742356128,6.92091963994));
#74228=CARTESIAN_POINT('Ctrl Pts',(5.94384247076,-42.6742356128,6.92091963994));
#74229=CARTESIAN_POINT('Ctrl Pts',(6.24384247076,-42.3742356128,7.75113701566));
#74230=CARTESIAN_POINT('Ctrl Pts',(6.24384247076,-42.4684833924,7.75113701566));
#74231=CARTESIAN_POINT('Ctrl Pts',(6.20683145426,-42.5627311721,7.74622965293));
#74232=CARTESIAN_POINT('Ctrl Pts',(6.13233802997,-42.6372245963,7.73635242463));
#74233=CARTESIAN_POINT('Ctrl Pts',(6.03809025037,-42.6742356128,7.72385592793));
#74234=CARTESIAN_POINT('Ctrl Pts',(5.94384247076,-42.6742356128,7.71135943123));
#74235=CARTESIAN_POINT('Ctrl Pts',(6.10624229678,-42.3742356128,8.58162297024));
#74236=CARTESIAN_POINT('Ctrl Pts',(6.10624229668,-42.4684833981,8.58162271341));
#74237=CARTESIAN_POINT('Ctrl Pts',(6.07004462212,-42.5627311834,8.5717822858));
#74238=CARTESIAN_POINT('Ctrl Pts',(5.99718824085,-42.6372246097,8.55197641205));
#74239=CARTESIAN_POINT('Ctrl Pts',(5.90501162182,-42.6742356217,8.52691852269));
#74240=CARTESIAN_POINT('Ctrl Pts',(5.81283500628,-42.6742356128,8.50186073478));
#74241=CARTESIAN_POINT('Ctrl Pts',(5.82995657026,-42.3742356128,9.38108114077));
#74242=CARTESIAN_POINT('Ctrl Pts',(5.82995672559,-42.4684833923,9.38108094408));
#74243=CARTESIAN_POINT('Ctrl Pts',(5.79540828589,-42.5627311717,9.36648855896));
#74244=CARTESIAN_POINT('Ctrl Pts',(5.72587117149,-42.6372245959,9.3371181729));
#74245=CARTESIAN_POINT('Ctrl Pts',(5.63789394152,-42.6742356126,9.29995939314));
#74246=CARTESIAN_POINT('Ctrl Pts',(5.54991664977,-42.6742356128,9.26280069107));
#74247=CARTESIAN_POINT('Ctrl Pts',(4.87592249919,-42.3742356128,11.1256648367));
#74248=CARTESIAN_POINT('Ctrl Pts',(4.87592228753,-42.4684833927,11.1256651047));
#74249=CARTESIAN_POINT('Ctrl Pts',(4.84702017121,-42.5627311725,11.1007324623));
#74250=CARTESIAN_POINT('Ctrl Pts',(4.78884811012,-42.6372245969,11.0505492956));
#74251=CARTESIAN_POINT('Ctrl Pts',(4.71524995296,-42.6742356132,10.9870582659));
#74252=CARTESIAN_POINT('Ctrl Pts',(4.64165187997,-42.6742356128,10.9235671304));
#74253=CARTESIAN_POINT('Ctrl Pts',(3.31613637806,-42.3742356128,12.395285601));
#74254=CARTESIAN_POINT('Ctrl Pts',(3.31613666647,-42.4684833921,12.3952852358));
#74255=CARTESIAN_POINT('Ctrl Pts',(3.29647895881,-42.5627311714,12.3628425782));
#74256=CARTESIAN_POINT('Ctrl Pts',(3.25691278652,-42.6372245955,12.2975445024));
#74257=CARTESIAN_POINT('Ctrl Pts',(3.20685419435,-42.6742356123,12.2149307397));
#74258=CARTESIAN_POINT('Ctrl Pts',(3.15679548747,-42.6742356128,12.1323171213));
#74259=CARTESIAN_POINT('Ctrl Pts',(2.26330649455,-42.3742356128,12.9089230556));
#74260=CARTESIAN_POINT('Ctrl Pts',(2.26330695882,-42.4684833774,12.9089230583));
#74261=CARTESIAN_POINT('Ctrl Pts',(2.24985627251,-42.5627311421,12.8734212448));
#74262=CARTESIAN_POINT('Ctrl Pts',(2.22278315419,-42.637224561,12.8019654469));
#74263=CARTESIAN_POINT('Ctrl Pts',(2.18853037756,-42.6742355893,12.7115608108));
#74264=CARTESIAN_POINT('Ctrl Pts',(2.15427741744,-42.6742356128,12.6211561643));
#74265=CARTESIAN_POINT('Ctrl Pts',(1.13128927566,-42.3742356128,13.1643460756));
#74266=CARTESIAN_POINT('Ctrl Pts',(1.13128927419,-42.4684833956,13.1643460756));
#74267=CARTESIAN_POINT('Ctrl Pts',(1.12462623999,-42.5627311784,13.127335058));
#74268=CARTESIAN_POINT('Ctrl Pts',(1.11121521855,-42.6372246038,13.0528416302));
#74269=CARTESIAN_POINT('Ctrl Pts',(1.09424786752,-42.6742356178,12.958593848));
#74270=CARTESIAN_POINT('Ctrl Pts',(1.07728051707,-42.6742356128,12.8643460678));
#74271=CARTESIAN_POINT('Ctrl Pts',(3.77707154442E-9,-42.3742356128,13.1643459857));
#74272=CARTESIAN_POINT('Ctrl Pts',(3.8111913625E-9,-42.4684833924,13.1643459857));
#74273=CARTESIAN_POINT('Ctrl Pts',(-1.41464807424E-7,-42.562731172,13.1273349695));
#74274=CARTESIAN_POINT('Ctrl Pts',(-4.33908818209E-7,-42.6372245963,13.0528415459));
#74275=CARTESIAN_POINT('Ctrl Pts',(-8.03924593562E-7,-42.6742356128,12.9585937671));
#74276=CARTESIAN_POINT('Ctrl Pts',(-1.17395376664E-6,-42.6742356128,12.8643459882));
#74277=CARTESIAN_POINT('',(6.24384247076,-42.3742356128,6.92091963994));
#74278=CARTESIAN_POINT('Origin',(5.94596376190762,-42.3763569039501,6.92091963994));
#74279=CARTESIAN_POINT('Ctrl Pts',(6.24384247076,-42.3742356128,6.92091963994));
#74280=CARTESIAN_POINT('Ctrl Pts',(6.24384247076,-42.3742356128,8.88234987966));
#74281=CARTESIAN_POINT('Ctrl Pts',(5.47580735138,-42.3742356128,10.8456101466));
#74282=CARTESIAN_POINT('Ctrl Pts',(3.92510661379,-42.3742356128,12.3963108842));
#74283=CARTESIAN_POINT('Ctrl Pts',(1.96184634686,-42.3742356128,13.1643460036));
#74284=CARTESIAN_POINT('Ctrl Pts',(3.5527136788E-15,-42.3742356128,13.1643460036));
#74285=CARTESIAN_POINT('Ctrl Pts',(5.55111512313E-15,-40.6742356128,13.1643460036));
#74286=CARTESIAN_POINT('Ctrl Pts',(5.55111512313E-15,-42.7142356128,13.1643460036));
#74287=CARTESIAN_POINT('Ctrl Pts',(1.96184634686,-40.6742356128,13.1643460036));
#74288=CARTESIAN_POINT('Ctrl Pts',(1.96184634686,-42.7142356128,13.1643460036));
#74289=CARTESIAN_POINT('Ctrl Pts',(3.92510661379,-40.6742356128,12.3963108842));
#74290=CARTESIAN_POINT('Ctrl Pts',(3.92510661379,-42.7142356128,12.3963108842));
#74291=CARTESIAN_POINT('Ctrl Pts',(5.47580735138,-40.6742356128,10.8456101466));
#74292=CARTESIAN_POINT('Ctrl Pts',(5.47580735138,-42.7142356128,10.8456101466));
#74293=CARTESIAN_POINT('Ctrl Pts',(6.24384247076,-40.6742356128,8.88234987966));
#74294=CARTESIAN_POINT('Ctrl Pts',(6.24384247076,-42.7142356128,8.88234987966));
#74295=CARTESIAN_POINT('Ctrl Pts',(6.24384247076,-40.6742356128,6.92091963994));
#74296=CARTESIAN_POINT('Ctrl Pts',(6.24384247076,-42.7142356128,6.92091963994));
#74297=CARTESIAN_POINT('',(6.24384247076,-41.5242356128,6.92091963994));
#74298=CARTESIAN_POINT('Origin',(5.94384247076,-42.3742356128,1.43032185727));
#74299=CARTESIAN_POINT('',(6.24384247076,-42.3742356128,5.17993069345));
#74300=CARTESIAN_POINT('Origin',(6.24384247076,-40.6742356128,6.92091963994));
#98283=UNCERTAINTY_MEASURE_WITH_UNIT(LENGTH_MEASURE(0.01),#98303,
'DISTANCE_ACCURACY_VALUE',
'Maximum model space distance between geometric entities at asserted c
onnectivities');
#98290=UNCERTAINTY_MEASURE_WITH_UNIT(LENGTH_MEASURE(0.01),#98303,
'DISTANCE_ACCURACY_VALUE',
'Maximum model space distance between geometric entities at asserted c
onnectivities');
#98295=(
GEOMETRIC_REPRESENTATION_CONTEXT(3)
GLOBAL_UNCERTAINTY_ASSIGNED_CONTEXT((#98283))
GLOBAL_UNIT_ASSIGNED_CONTEXT((#98303,#98305,#98306))
REPRESENTATION_CONTEXT('','3D')
);
#98302=(
GEOMETRIC_REPRESENTATION_CONTEXT(3)
GLOBAL_UNCERTAINTY_ASSIGNED_CONTEXT((#98290))
GLOBAL_UNIT_ASSIGNED_CONTEXT((#98303,#98305,#98306))
REPRESENTATION_CONTEXT('','3D')
);
#98303=(
LENGTH_UNIT()
NAMED_UNIT(*)
SI_UNIT(.MILLI.,.METRE.)
);
#98305=(
NAMED_UNIT(*)
PLANE_ANGLE_UNIT()
SI_UNIT($,.RADIAN.)
);
#98306=(
NAMED_UNIT(*)
SI_UNIT($,.STERADIAN.)
SOLID_ANGLE_UNIT()
);
#98311=SHAPE_DEFINITION_REPRESENTATION(#98322,#98343);
#98322=PRODUCT_DEFINITION_SHAPE('',$,#98355);
#98343=SHAPE_REPRESENTATION('',(#34920),#98295);
#98350=PRODUCT_DEFINITION_CONTEXT('part definition',#98385,'design');
#98355=PRODUCT_DEFINITION('Bottom Gaskets','Bottom Gaskets',#98366,#98350);
#98366=PRODUCT_DEFINITION_FORMATION('',$,#98391);
#98385=APPLICATION_CONTEXT(
'Core Data for Automotive Mechanical Design Process');
#98386=PRODUCT_CONTEXT('part definition',#98385,'mechanical');
#98391=PRODUCT('Bottom Gaskets','Bottom Gaskets',$,(#98386));
#98399=PRESENTATION_STYLE_ASSIGNMENT((#98401));
#98401=SURFACE_STYLE_USAGE(.BOTH.,#98403);
#98403=SURFACE_SIDE_STYLE('',(#98405));
#98405=SURFACE_STYLE_FILL_AREA(#98407);
#98407=FILL_AREA_STYLE('Opaque(202,209,238)',(#98409));
#98409=FILL_AREA_STYLE_COLOUR('Opaque(202,209,238)',#98411);
#98411=COLOUR_RGB('Opaque(202,209,238)', 0.31764706, 0.68627451, 0.89019608);
ENDSEC;
END-ISO-10303-21;
